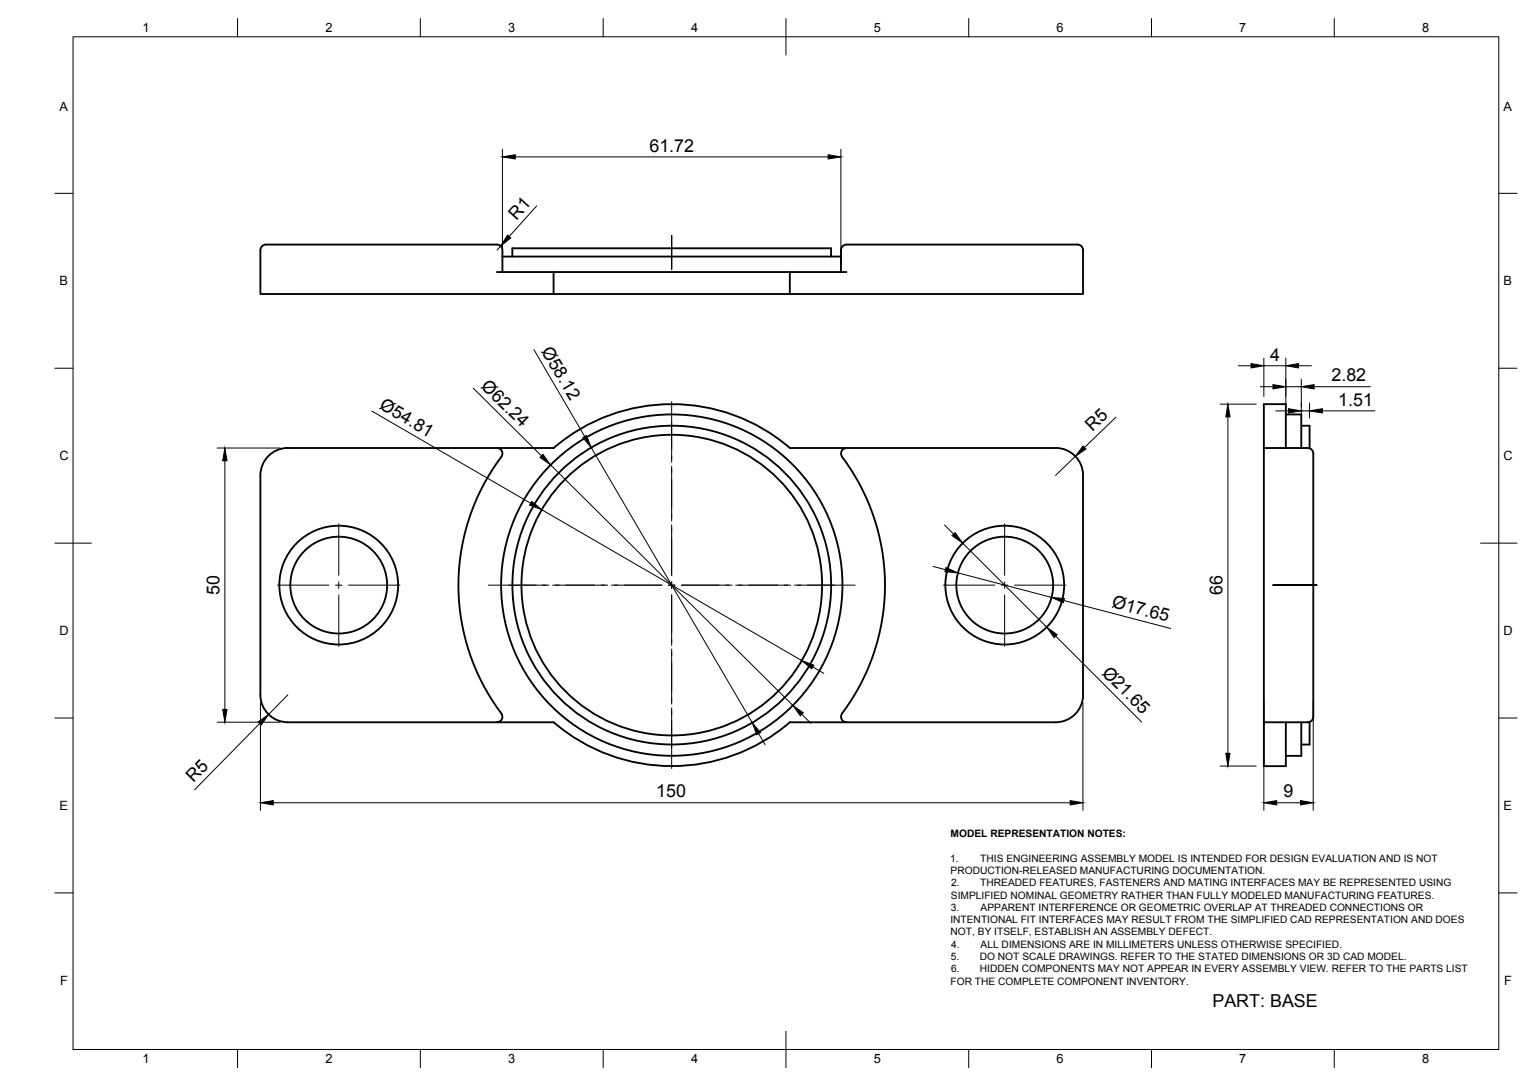
ISO-10303-21;
HEADER;
/* Generated by software containing ST-Developer
 * from STEP Tools, Inc. (www.steptools.com) 
 */

FILE_DESCRIPTION(
/* description */ (''),
/* implementation_level */ '2;1');

FILE_NAME(
/* name */ 'Base.step',
/* time_stamp */ '2026-10-04T22:47:03-07:00',
/* author */ (''),
/* organization */ (''),
/* preprocessor_version */ 'ST-DEVELOPER v20.2',
/* originating_system */ 'Autodesk Translation Framework v15.15.0.0',
/* authorisation */ '');

FILE_SCHEMA (('AUTOMOTIVE_DESIGN { 1 0 10303 214 3 1 1 }'));
ENDSEC;

DATA;
#10=MECHANICAL_DESIGN_GEOMETRIC_PRESENTATION_REPRESENTATION('',(#82),#19878);
#39=SPHERICAL_SURFACE('',#5318,1.);
#40=SPHERICAL_SURFACE('',#5323,1.);
#41=SPHERICAL_SURFACE('',#5367,1.);
#42=SPHERICAL_SURFACE('',#5372,1.);
#50=TOROIDAL_SURFACE('',#5313,39.889325151227,1.);
#51=TOROIDAL_SURFACE('',#5335,4.,1.);
#52=TOROIDAL_SURFACE('',#5340,4.,1.);
#53=TOROIDAL_SURFACE('',#5362,39.889325151227,1.);
#54=TOROIDAL_SURFACE('',#5384,4.,1.);
#55=TOROIDAL_SURFACE('',#5389,4.,1.);
#61=CONICAL_SURFACE('',#5342,9.8273485245745,0.785398163397449);
#62=CONICAL_SURFACE('',#5391,9.8273485245745,0.785398163397449);
#68=SHAPE_REPRESENTATION_RELATIONSHIP('SRR','None',#19912,#75);
#75=ADVANCED_BREP_SHAPE_REPRESENTATION('',(#89),#19876);
#82=STYLED_ITEM('',(#19951),#89);
#89=MANIFOLD_SOLID_BREP('Body1',#4830);
#104=FACE_BOUND('',#849,.T.);
#105=FACE_BOUND('',#871,.T.);
#106=FACE_BOUND('',#886,.T.);
#107=FACE_BOUND('',#887,.T.);
#108=FACE_BOUND('',#889,.T.);
#109=FACE_BOUND('',#892,.T.);
#110=FACE_BOUND('',#895,.T.);
#312=PLANE('',#5325);
#313=PLANE('',#5328);
#314=PLANE('',#5334);
#315=PLANE('',#5348);
#316=PLANE('',#5374);
#317=PLANE('',#5377);
#318=PLANE('',#5383);
#319=PLANE('',#5397);
#320=PLANE('',#5405);
#321=PLANE('',#5406);
#322=PLANE('',#5407);
#323=PLANE('',#5411);
#324=PLANE('',#5415);
#552=FACE_OUTER_BOUND('',#841,.T.);
#553=FACE_OUTER_BOUND('',#842,.T.);
#554=FACE_OUTER_BOUND('',#843,.T.);
#555=FACE_OUTER_BOUND('',#844,.T.);
#556=FACE_OUTER_BOUND('',#845,.T.);
#557=FACE_OUTER_BOUND('',#846,.T.);
#558=FACE_OUTER_BOUND('',#847,.T.);
#559=FACE_OUTER_BOUND('',#848,.T.);
#560=FACE_OUTER_BOUND('',#850,.T.);
#561=FACE_OUTER_BOUND('',#851,.T.);
#562=FACE_OUTER_BOUND('',#852,.T.);
#563=FACE_OUTER_BOUND('',#853,.T.);
#564=FACE_OUTER_BOUND('',#854,.T.);
#565=FACE_OUTER_BOUND('',#855,.T.);
#566=FACE_OUTER_BOUND('',#856,.T.);
#567=FACE_OUTER_BOUND('',#857,.T.);
#568=FACE_OUTER_BOUND('',#858,.T.);
#569=FACE_OUTER_BOUND('',#859,.T.);
#570=FACE_OUTER_BOUND('',#860,.T.);
#571=FACE_OUTER_BOUND('',#861,.T.);
#572=FACE_OUTER_BOUND('',#862,.T.);
#573=FACE_OUTER_BOUND('',#863,.T.);
#574=FACE_OUTER_BOUND('',#864,.T.);
#575=FACE_OUTER_BOUND('',#865,.T.);
#576=FACE_OUTER_BOUND('',#866,.T.);
#577=FACE_OUTER_BOUND('',#867,.T.);
#578=FACE_OUTER_BOUND('',#868,.T.);
#579=FACE_OUTER_BOUND('',#869,.T.);
#580=FACE_OUTER_BOUND('',#870,.T.);
#581=FACE_OUTER_BOUND('',#872,.T.);
#582=FACE_OUTER_BOUND('',#873,.T.);
#583=FACE_OUTER_BOUND('',#874,.T.);
#584=FACE_OUTER_BOUND('',#875,.T.);
#585=FACE_OUTER_BOUND('',#876,.T.);
#586=FACE_OUTER_BOUND('',#877,.T.);
#587=FACE_OUTER_BOUND('',#878,.T.);
#588=FACE_OUTER_BOUND('',#879,.T.);
#589=FACE_OUTER_BOUND('',#880,.T.);
#590=FACE_OUTER_BOUND('',#881,.T.);
#591=FACE_OUTER_BOUND('',#882,.T.);
#592=FACE_OUTER_BOUND('',#883,.T.);
#593=FACE_OUTER_BOUND('',#884,.T.);
#594=FACE_OUTER_BOUND('',#885,.T.);
#595=FACE_OUTER_BOUND('',#888,.T.);
#596=FACE_OUTER_BOUND('',#890,.T.);
#597=FACE_OUTER_BOUND('',#891,.T.);
#598=FACE_OUTER_BOUND('',#893,.T.);
#599=FACE_OUTER_BOUND('',#894,.T.);
#841=EDGE_LOOP('',(#4213,#4214,#4215,#4216));
#842=EDGE_LOOP('',(#4217,#4218,#4219,#4220));
#843=EDGE_LOOP('',(#4221,#4222,#4223));
#844=EDGE_LOOP('',(#4224,#4225,#4226,#4227));
#845=EDGE_LOOP('',(#4228,#4229,#4230));
#846=EDGE_LOOP('',(#4231,#4232,#4233,#4234,#4235,#4236));
#847=EDGE_LOOP('',(#4237,#4238,#4239,#4240));
#848=EDGE_LOOP('',(#4241,#4242,#4243,#4244,#4245,#4246));
#849=EDGE_LOOP('',(#4247));
#850=EDGE_LOOP('',(#4248,#4249,#4250,#4251));
#851=EDGE_LOOP('',(#4252,#4253,#4254,#4255,#4256,#4257));
#852=EDGE_LOOP('',(#4258,#4259,#4260,#4261));
#853=EDGE_LOOP('',(#4262,#4263,#4264,#4265));
#854=EDGE_LOOP('',(#4266,#4267,#4268,#4269));
#855=EDGE_LOOP('',(#4270,#4271,#4272,#4273));
#856=EDGE_LOOP('',(#4274,#4275,#4276,#4277));
#857=EDGE_LOOP('',(#4278,#4279,#4280,#4281));
#858=EDGE_LOOP('',(#4282,#4283,#4284,#4285));
#859=EDGE_LOOP('',(#4286,#4287,#4288,#4289));
#860=EDGE_LOOP('',(#4290,#4291,#4292,#4293));
#861=EDGE_LOOP('',(#4294,#4295,#4296,#4297));
#862=EDGE_LOOP('',(#4298,#4299,#4300,#4301));
#863=EDGE_LOOP('',(#4302,#4303,#4304,#4305));
#864=EDGE_LOOP('',(#4306,#4307,#4308,#4309));
#865=EDGE_LOOP('',(#4310,#4311,#4312));
#866=EDGE_LOOP('',(#4313,#4314,#4315,#4316));
#867=EDGE_LOOP('',(#4317,#4318,#4319));
#868=EDGE_LOOP('',(#4320,#4321,#4322,#4323,#4324,#4325));
#869=EDGE_LOOP('',(#4326,#4327,#4328,#4329));
#870=EDGE_LOOP('',(#4330,#4331,#4332,#4333,#4334,#4335));
#871=EDGE_LOOP('',(#4336));
#872=EDGE_LOOP('',(#4337,#4338,#4339,#4340));
#873=EDGE_LOOP('',(#4341,#4342,#4343,#4344,#4345,#4346));
#874=EDGE_LOOP('',(#4347,#4348,#4349,#4350));
#875=EDGE_LOOP('',(#4351,#4352,#4353,#4354));
#876=EDGE_LOOP('',(#4355,#4356,#4357,#4358));
#877=EDGE_LOOP('',(#4359,#4360,#4361,#4362));
#878=EDGE_LOOP('',(#4363,#4364,#4365,#4366));
#879=EDGE_LOOP('',(#4367,#4368,#4369,#4370));
#880=EDGE_LOOP('',(#4371,#4372,#4373,#4374));
#881=EDGE_LOOP('',(#4375,#4376,#4377,#4378));
#882=EDGE_LOOP('',(#4379,#4380,#4381,#4382));
#883=EDGE_LOOP('',(#4383,#4384,#4385,#4386));
#884=EDGE_LOOP('',(#4387));
#885=EDGE_LOOP('',(#4388,#4389,#4390,#4391,#4392,#4393,#4394,#4395,#4396,
#4397,#4398,#4399));
#886=EDGE_LOOP('',(#4400));
#887=EDGE_LOOP('',(#4401));
#888=EDGE_LOOP('',(#4402,#4403,#4404,#4405,#4406,#4407,#4408,#4409,#4410,
#4411,#4412,#4413));
#889=EDGE_LOOP('',(#4414));
#890=EDGE_LOOP('',(#4415,#4416,#4417,#4418));
#891=EDGE_LOOP('',(#4419));
#892=EDGE_LOOP('',(#4420));
#893=EDGE_LOOP('',(#4421,#4422,#4423,#4424));
#894=EDGE_LOOP('',(#4425));
#895=EDGE_LOOP('',(#4426));
#1204=LINE('',#19635,#1560);
#1205=LINE('',#19638,#1561);
#1206=LINE('',#19653,#1562);
#1207=LINE('',#19656,#1563);
#1208=LINE('',#19661,#1564);
#1209=LINE('',#19663,#1565);
#1210=LINE('',#19665,#1566);
#1211=LINE('',#19667,#1567);
#1212=LINE('',#19668,#1568);
#1213=LINE('',#19672,#1569);
#1214=LINE('',#19677,#1570);
#1215=LINE('',#19680,#1571);
#1216=LINE('',#19686,#1572);
#1217=LINE('',#19689,#1573);
#1218=LINE('',#19691,#1574);
#1219=LINE('',#19693,#1575);
#1220=LINE('',#19694,#1576);
#1221=LINE('',#19702,#1577);
#1222=LINE('',#19708,#1578);
#1223=LINE('',#19712,#1579);
#1224=LINE('',#19716,#1580);
#1225=LINE('',#19719,#1581);
#1226=LINE('',#19720,#1582);
#1227=LINE('',#19729,#1583);
#1228=LINE('',#19735,#1584);
#1229=LINE('',#19742,#1585);
#1230=LINE('',#19745,#1586);
#1231=LINE('',#19760,#1587);
#1232=LINE('',#19763,#1588);
#1233=LINE('',#19767,#1589);
#1234=LINE('',#19769,#1590);
#1235=LINE('',#19771,#1591);
#1236=LINE('',#19772,#1592);
#1237=LINE('',#19775,#1593);
#1238=LINE('',#19779,#1594);
#1239=LINE('',#19783,#1595);
#1240=LINE('',#19789,#1596);
#1241=LINE('',#19792,#1597);
#1242=LINE('',#19794,#1598);
#1243=LINE('',#19795,#1599);
#1244=LINE('',#19803,#1600);
#1245=LINE('',#19809,#1601);
#1246=LINE('',#19812,#1602);
#1247=LINE('',#19816,#1603);
#1248=LINE('',#19820,#1604);
#1249=LINE('',#19821,#1605);
#1250=LINE('',#19830,#1606);
#1251=LINE('',#19840,#1607);
#1252=LINE('',#19847,#1608);
#1560=VECTOR('',#6538,10.);
#1561=VECTOR('',#6541,10.);
#1562=VECTOR('',#6560,10.);
#1563=VECTOR('',#6563,10.);
#1564=VECTOR('',#6570,10.);
#1565=VECTOR('',#6571,10.);
#1566=VECTOR('',#6572,10.);
#1567=VECTOR('',#6573,10.);
#1568=VECTOR('',#6574,10.);
#1569=VECTOR('',#6579,10.);
#1570=VECTOR('',#6584,10.);
#1571=VECTOR('',#6587,10.);
#1572=VECTOR('',#6594,10.);
#1573=VECTOR('',#6597,10.);
#1574=VECTOR('',#6598,10.);
#1575=VECTOR('',#6599,10.);
#1576=VECTOR('',#6600,10.);
#1577=VECTOR('',#6611,10.);
#1578=VECTOR('',#6620,9.8273485245745);
#1579=VECTOR('',#6625,8.8273485245745);
#1580=VECTOR('',#6630,10.);
#1581=VECTOR('',#6633,10.);
#1582=VECTOR('',#6634,10.);
#1583=VECTOR('',#6647,10.);
#1584=VECTOR('',#6654,10.);
#1585=VECTOR('',#6661,10.);
#1586=VECTOR('',#6664,10.);
#1587=VECTOR('',#6683,10.);
#1588=VECTOR('',#6686,10.);
#1589=VECTOR('',#6693,10.);
#1590=VECTOR('',#6694,10.);
#1591=VECTOR('',#6695,10.);
#1592=VECTOR('',#6696,10.);
#1593=VECTOR('',#6699,10.);
#1594=VECTOR('',#6704,10.);
#1595=VECTOR('',#6707,10.);
#1596=VECTOR('',#6714,10.);
#1597=VECTOR('',#6719,10.);
#1598=VECTOR('',#6720,10.);
#1599=VECTOR('',#6721,10.);
#1600=VECTOR('',#6732,10.);
#1601=VECTOR('',#6741,9.8273485245745);
#1602=VECTOR('',#6744,8.8273485245745);
#1603=VECTOR('',#6749,10.);
#1604=VECTOR('',#6754,10.);
#1605=VECTOR('',#6755,10.);
#1606=VECTOR('',#6768,27.4027293621977);
#1607=VECTOR('',#6783,31.1192710879259);
#1608=VECTOR('',#6792,29.0578798664922);
#1815=CIRCLE('',#5311,0.999999999999996);
#1816=CIRCLE('',#5312,1.);
#1817=CIRCLE('',#5314,0.999999999999999);
#1818=CIRCLE('',#5315,38.889325151227);
#1819=CIRCLE('',#5316,1.);
#1820=CIRCLE('',#5317,39.889325151227);
#1821=CIRCLE('',#5319,1.);
#1822=CIRCLE('',#5321,1.);
#1823=CIRCLE('',#5322,1.);
#1824=CIRCLE('',#5324,1.);
#1825=CIRCLE('',#5327,1.);
#1826=CIRCLE('',#5329,4.);
#1827=CIRCLE('',#5330,4.);
#1828=CIRCLE('',#5331,10.8273485245745);
#1829=CIRCLE('',#5333,1.);
#1830=CIRCLE('',#5336,1.);
#1831=CIRCLE('',#5337,5.);
#1832=CIRCLE('',#5339,1.);
#1833=CIRCLE('',#5341,5.);
#1834=CIRCLE('',#5343,8.8273485245745);
#1835=CIRCLE('',#5345,8.8273485245745);
#1836=CIRCLE('',#5347,5.);
#1837=CIRCLE('',#5350,5.);
#1838=CIRCLE('',#5352,38.889325151227);
#1839=CIRCLE('',#5354,33.);
#1840=CIRCLE('',#5355,33.);
#1841=CIRCLE('',#5357,33.);
#1842=CIRCLE('',#5358,33.);
#1843=CIRCLE('',#5360,0.999999999999996);
#1844=CIRCLE('',#5361,1.);
#1845=CIRCLE('',#5363,0.999999999999999);
#1846=CIRCLE('',#5364,39.889325151227);
#1847=CIRCLE('',#5365,1.);
#1848=CIRCLE('',#5366,38.889325151227);
#1849=CIRCLE('',#5368,1.);
#1850=CIRCLE('',#5370,1.);
#1851=CIRCLE('',#5371,1.);
#1852=CIRCLE('',#5373,1.);
#1853=CIRCLE('',#5376,1.);
#1854=CIRCLE('',#5378,4.);
#1855=CIRCLE('',#5379,4.);
#1856=CIRCLE('',#5380,10.8273485245745);
#1857=CIRCLE('',#5382,1.);
#1858=CIRCLE('',#5385,1.);
#1859=CIRCLE('',#5386,5.);
#1860=CIRCLE('',#5388,1.);
#1861=CIRCLE('',#5390,5.);
#1862=CIRCLE('',#5392,8.8273485245745);
#1863=CIRCLE('',#5394,8.8273485245745);
#1864=CIRCLE('',#5396,5.);
#1865=CIRCLE('',#5399,5.);
#1866=CIRCLE('',#5401,38.889325151227);
#1867=CIRCLE('',#5403,27.4027293621977);
#1868=CIRCLE('',#5404,27.4027293621977);
#1869=CIRCLE('',#5408,31.1192710879259);
#1870=CIRCLE('',#5410,31.1192710879259);
#1871=CIRCLE('',#5412,29.0578798664922);
#1872=CIRCLE('',#5414,29.0578798664922);
#2260=VERTEX_POINT('',#19631);
#2261=VERTEX_POINT('',#19632);
#2262=VERTEX_POINT('',#19634);
#2263=VERTEX_POINT('',#19636);
#2264=VERTEX_POINT('',#19640);
#2265=VERTEX_POINT('',#19641);
#2266=VERTEX_POINT('',#19644);
#2267=VERTEX_POINT('',#19650);
#2268=VERTEX_POINT('',#19652);
#2269=VERTEX_POINT('',#19654);
#2270=VERTEX_POINT('',#19660);
#2271=VERTEX_POINT('',#19662);
#2272=VERTEX_POINT('',#19664);
#2273=VERTEX_POINT('',#19666);
#2274=VERTEX_POINT('',#19670);
#2275=VERTEX_POINT('',#19674);
#2276=VERTEX_POINT('',#19676);
#2277=VERTEX_POINT('',#19678);
#2278=VERTEX_POINT('',#19681);
#2279=VERTEX_POINT('',#19684);
#2280=VERTEX_POINT('',#19688);
#2281=VERTEX_POINT('',#19690);
#2282=VERTEX_POINT('',#19692);
#2283=VERTEX_POINT('',#19696);
#2284=VERTEX_POINT('',#19700);
#2285=VERTEX_POINT('',#19706);
#2286=VERTEX_POINT('',#19710);
#2287=VERTEX_POINT('',#19714);
#2288=VERTEX_POINT('',#19718);
#2289=VERTEX_POINT('',#19726);
#2290=VERTEX_POINT('',#19728);
#2291=VERTEX_POINT('',#19732);
#2292=VERTEX_POINT('',#19734);
#2293=VERTEX_POINT('',#19738);
#2294=VERTEX_POINT('',#19739);
#2295=VERTEX_POINT('',#19741);
#2296=VERTEX_POINT('',#19743);
#2297=VERTEX_POINT('',#19747);
#2298=VERTEX_POINT('',#19748);
#2299=VERTEX_POINT('',#19750);
#2300=VERTEX_POINT('',#19757);
#2301=VERTEX_POINT('',#19759);
#2302=VERTEX_POINT('',#19761);
#2303=VERTEX_POINT('',#19768);
#2304=VERTEX_POINT('',#19770);
#2305=VERTEX_POINT('',#19774);
#2306=VERTEX_POINT('',#19778);
#2307=VERTEX_POINT('',#19780);
#2308=VERTEX_POINT('',#19782);
#2309=VERTEX_POINT('',#19785);
#2310=VERTEX_POINT('',#19788);
#2311=VERTEX_POINT('',#19793);
#2312=VERTEX_POINT('',#19797);
#2313=VERTEX_POINT('',#19801);
#2314=VERTEX_POINT('',#19807);
#2315=VERTEX_POINT('',#19811);
#2316=VERTEX_POINT('',#19815);
#2317=VERTEX_POINT('',#19819);
#2318=VERTEX_POINT('',#19827);
#2319=VERTEX_POINT('',#19829);
#2320=VERTEX_POINT('',#19835);
#2321=VERTEX_POINT('',#19838);
#2322=VERTEX_POINT('',#19842);
#2323=VERTEX_POINT('',#19845);
#2918=EDGE_CURVE('',#2260,#2261,#1815,.T.);
#2919=EDGE_CURVE('',#2262,#2260,#1204,.T.);
#2920=EDGE_CURVE('',#2263,#2262,#1816,.F.);
#2921=EDGE_CURVE('',#2261,#2263,#1205,.T.);
#2922=EDGE_CURVE('',#2264,#2265,#1817,.T.);
#2923=EDGE_CURVE('',#2260,#2264,#1818,.T.);
#2924=EDGE_CURVE('',#2266,#2260,#1819,.T.);
#2925=EDGE_CURVE('',#2265,#2266,#1820,.T.);
#2926=EDGE_CURVE('',#2266,#2261,#1821,.T.);
#2927=EDGE_CURVE('',#2267,#2264,#1822,.T.);
#2928=EDGE_CURVE('',#2268,#2267,#1206,.T.);
#2929=EDGE_CURVE('',#2269,#2268,#1823,.F.);
#2930=EDGE_CURVE('',#2264,#2269,#1207,.T.);
#2931=EDGE_CURVE('',#2267,#2265,#1824,.T.);
#2932=EDGE_CURVE('',#2270,#2263,#1208,.T.);
#2933=EDGE_CURVE('',#2271,#2270,#1209,.T.);
#2934=EDGE_CURVE('',#2271,#2272,#1210,.T.);
#2935=EDGE_CURVE('',#2272,#2273,#1211,.T.);
#2936=EDGE_CURVE('',#2273,#2261,#1212,.T.);
#2937=EDGE_CURVE('',#2274,#2273,#1825,.T.);
#2938=EDGE_CURVE('',#2266,#2274,#1213,.T.);
#2939=EDGE_CURVE('',#2274,#2275,#1826,.T.);
#2940=EDGE_CURVE('',#2275,#2276,#1214,.T.);
#2941=EDGE_CURVE('',#2276,#2277,#1827,.T.);
#2942=EDGE_CURVE('',#2277,#2265,#1215,.T.);
#2943=EDGE_CURVE('',#2278,#2278,#1828,.T.);
#2944=EDGE_CURVE('',#2277,#2279,#1829,.T.);
#2945=EDGE_CURVE('',#2267,#2279,#1216,.T.);
#2946=EDGE_CURVE('',#2279,#2280,#1217,.T.);
#2947=EDGE_CURVE('',#2280,#2281,#1218,.T.);
#2948=EDGE_CURVE('',#2282,#2281,#1219,.T.);
#2949=EDGE_CURVE('',#2268,#2282,#1220,.T.);
#2950=EDGE_CURVE('',#2275,#2283,#1830,.T.);
#2951=EDGE_CURVE('',#2283,#2273,#1831,.T.);
#2952=EDGE_CURVE('',#2276,#2284,#1832,.T.);
#2953=EDGE_CURVE('',#2284,#2283,#1221,.T.);
#2954=EDGE_CURVE('',#2279,#2284,#1833,.T.);
#2955=EDGE_CURVE('',#2285,#2285,#1834,.T.);
#2956=EDGE_CURVE('',#2285,#2278,#1222,.T.);
#2957=EDGE_CURVE('',#2286,#2286,#1835,.T.);
#2958=EDGE_CURVE('',#2286,#2285,#1223,.T.);
#2959=EDGE_CURVE('',#2287,#2272,#1836,.T.);
#2960=EDGE_CURVE('',#2283,#2287,#1224,.T.);
#2961=EDGE_CURVE('',#2287,#2288,#1225,.T.);
#2962=EDGE_CURVE('',#2288,#2284,#1226,.T.);
#2963=EDGE_CURVE('',#2280,#2288,#1837,.T.);
#2964=EDGE_CURVE('',#2262,#2269,#1838,.T.);
#2965=EDGE_CURVE('',#2281,#2289,#1839,.F.);
#2966=EDGE_CURVE('',#2289,#2290,#1227,.T.);
#2967=EDGE_CURVE('',#2282,#2290,#1840,.T.);
#2968=EDGE_CURVE('',#2291,#2270,#1841,.T.);
#2969=EDGE_CURVE('',#2291,#2292,#1228,.T.);
#2970=EDGE_CURVE('',#2292,#2271,#1842,.F.);
#2971=EDGE_CURVE('',#2293,#2294,#1843,.T.);
#2972=EDGE_CURVE('',#2294,#2295,#1229,.T.);
#2973=EDGE_CURVE('',#2295,#2296,#1844,.F.);
#2974=EDGE_CURVE('',#2296,#2293,#1230,.T.);
#2975=EDGE_CURVE('',#2297,#2298,#1845,.T.);
#2976=EDGE_CURVE('',#2298,#2299,#1846,.T.);
#2977=EDGE_CURVE('',#2299,#2293,#1847,.T.);
#2978=EDGE_CURVE('',#2293,#2297,#1848,.T.);
#2979=EDGE_CURVE('',#2299,#2294,#1849,.T.);
#2980=EDGE_CURVE('',#2300,#2297,#1850,.T.);
#2981=EDGE_CURVE('',#2297,#2301,#1231,.T.);
#2982=EDGE_CURVE('',#2301,#2302,#1851,.F.);
#2983=EDGE_CURVE('',#2302,#2300,#1232,.T.);
#2984=EDGE_CURVE('',#2300,#2298,#1852,.T.);
#2985=EDGE_CURVE('',#2291,#2295,#1233,.T.);
#2986=EDGE_CURVE('',#2303,#2294,#1234,.T.);
#2987=EDGE_CURVE('',#2304,#2303,#1235,.T.);
#2988=EDGE_CURVE('',#2292,#2304,#1236,.T.);
#2989=EDGE_CURVE('',#2299,#2305,#1237,.T.);
#2990=EDGE_CURVE('',#2305,#2303,#1853,.T.);
#2991=EDGE_CURVE('',#2306,#2298,#1238,.T.);
#2992=EDGE_CURVE('',#2307,#2306,#1854,.T.);
#2993=EDGE_CURVE('',#2308,#2307,#1239,.T.);
#2994=EDGE_CURVE('',#2305,#2308,#1855,.T.);
#2995=EDGE_CURVE('',#2309,#2309,#1856,.T.);
#2996=EDGE_CURVE('',#2300,#2310,#1240,.T.);
#2997=EDGE_CURVE('',#2306,#2310,#1857,.T.);
#2998=EDGE_CURVE('',#2302,#2290,#1241,.T.);
#2999=EDGE_CURVE('',#2311,#2289,#1242,.T.);
#3000=EDGE_CURVE('',#2310,#2311,#1243,.T.);
#3001=EDGE_CURVE('',#2308,#2312,#1858,.T.);
#3002=EDGE_CURVE('',#2312,#2303,#1859,.T.);
#3003=EDGE_CURVE('',#2307,#2313,#1860,.T.);
#3004=EDGE_CURVE('',#2313,#2312,#1244,.T.);
#3005=EDGE_CURVE('',#2310,#2313,#1861,.T.);
#3006=EDGE_CURVE('',#2314,#2314,#1862,.T.);
#3007=EDGE_CURVE('',#2314,#2309,#1245,.T.);
#3008=EDGE_CURVE('',#2314,#2315,#1246,.T.);
#3009=EDGE_CURVE('',#2315,#2315,#1863,.T.);
#3010=EDGE_CURVE('',#2312,#2316,#1247,.T.);
#3011=EDGE_CURVE('',#2316,#2304,#1864,.T.);
#3012=EDGE_CURVE('',#2317,#2313,#1248,.T.);
#3013=EDGE_CURVE('',#2316,#2317,#1249,.T.);
#3014=EDGE_CURVE('',#2311,#2317,#1865,.T.);
#3015=EDGE_CURVE('',#2296,#2301,#1866,.T.);
#3016=EDGE_CURVE('',#2318,#2318,#1867,.T.);
#3017=EDGE_CURVE('',#2318,#2319,#1250,.T.);
#3018=EDGE_CURVE('',#2319,#2319,#1868,.T.);
#3019=EDGE_CURVE('',#2320,#2320,#1869,.T.);
#3020=EDGE_CURVE('',#2321,#2321,#1870,.T.);
#3021=EDGE_CURVE('',#2321,#2320,#1251,.T.);
#3022=EDGE_CURVE('',#2322,#2322,#1871,.T.);
#3023=EDGE_CURVE('',#2323,#2323,#1872,.T.);
#3024=EDGE_CURVE('',#2323,#2322,#1252,.T.);
#4213=ORIENTED_EDGE('',*,*,#2918,.F.);
#4214=ORIENTED_EDGE('',*,*,#2919,.F.);
#4215=ORIENTED_EDGE('',*,*,#2920,.F.);
#4216=ORIENTED_EDGE('',*,*,#2921,.F.);
#4217=ORIENTED_EDGE('',*,*,#2922,.F.);
#4218=ORIENTED_EDGE('',*,*,#2923,.F.);
#4219=ORIENTED_EDGE('',*,*,#2924,.F.);
#4220=ORIENTED_EDGE('',*,*,#2925,.F.);
#4221=ORIENTED_EDGE('',*,*,#2924,.T.);
#4222=ORIENTED_EDGE('',*,*,#2918,.T.);
#4223=ORIENTED_EDGE('',*,*,#2926,.F.);
#4224=ORIENTED_EDGE('',*,*,#2927,.F.);
#4225=ORIENTED_EDGE('',*,*,#2928,.F.);
#4226=ORIENTED_EDGE('',*,*,#2929,.F.);
#4227=ORIENTED_EDGE('',*,*,#2930,.F.);
#4228=ORIENTED_EDGE('',*,*,#2927,.T.);
#4229=ORIENTED_EDGE('',*,*,#2922,.T.);
#4230=ORIENTED_EDGE('',*,*,#2931,.F.);
#4231=ORIENTED_EDGE('',*,*,#2932,.F.);
#4232=ORIENTED_EDGE('',*,*,#2933,.F.);
#4233=ORIENTED_EDGE('',*,*,#2934,.T.);
#4234=ORIENTED_EDGE('',*,*,#2935,.T.);
#4235=ORIENTED_EDGE('',*,*,#2936,.T.);
#4236=ORIENTED_EDGE('',*,*,#2921,.T.);
#4237=ORIENTED_EDGE('',*,*,#2926,.T.);
#4238=ORIENTED_EDGE('',*,*,#2936,.F.);
#4239=ORIENTED_EDGE('',*,*,#2937,.F.);
#4240=ORIENTED_EDGE('',*,*,#2938,.F.);
#4241=ORIENTED_EDGE('',*,*,#2925,.T.);
#4242=ORIENTED_EDGE('',*,*,#2938,.T.);
#4243=ORIENTED_EDGE('',*,*,#2939,.T.);
#4244=ORIENTED_EDGE('',*,*,#2940,.T.);
#4245=ORIENTED_EDGE('',*,*,#2941,.T.);
#4246=ORIENTED_EDGE('',*,*,#2942,.T.);
#4247=ORIENTED_EDGE('',*,*,#2943,.T.);
#4248=ORIENTED_EDGE('',*,*,#2931,.T.);
#4249=ORIENTED_EDGE('',*,*,#2942,.F.);
#4250=ORIENTED_EDGE('',*,*,#2944,.T.);
#4251=ORIENTED_EDGE('',*,*,#2945,.F.);
#4252=ORIENTED_EDGE('',*,*,#2928,.T.);
#4253=ORIENTED_EDGE('',*,*,#2945,.T.);
#4254=ORIENTED_EDGE('',*,*,#2946,.T.);
#4255=ORIENTED_EDGE('',*,*,#2947,.T.);
#4256=ORIENTED_EDGE('',*,*,#2948,.F.);
#4257=ORIENTED_EDGE('',*,*,#2949,.F.);
#4258=ORIENTED_EDGE('',*,*,#2950,.F.);
#4259=ORIENTED_EDGE('',*,*,#2939,.F.);
#4260=ORIENTED_EDGE('',*,*,#2937,.T.);
#4261=ORIENTED_EDGE('',*,*,#2951,.F.);
#4262=ORIENTED_EDGE('',*,*,#2952,.F.);
#4263=ORIENTED_EDGE('',*,*,#2940,.F.);
#4264=ORIENTED_EDGE('',*,*,#2950,.T.);
#4265=ORIENTED_EDGE('',*,*,#2953,.F.);
#4266=ORIENTED_EDGE('',*,*,#2944,.F.);
#4267=ORIENTED_EDGE('',*,*,#2941,.F.);
#4268=ORIENTED_EDGE('',*,*,#2952,.T.);
#4269=ORIENTED_EDGE('',*,*,#2954,.F.);
#4270=ORIENTED_EDGE('',*,*,#2955,.F.);
#4271=ORIENTED_EDGE('',*,*,#2956,.T.);
#4272=ORIENTED_EDGE('',*,*,#2943,.F.);
#4273=ORIENTED_EDGE('',*,*,#2956,.F.);
#4274=ORIENTED_EDGE('',*,*,#2957,.T.);
#4275=ORIENTED_EDGE('',*,*,#2958,.T.);
#4276=ORIENTED_EDGE('',*,*,#2955,.T.);
#4277=ORIENTED_EDGE('',*,*,#2958,.F.);
#4278=ORIENTED_EDGE('',*,*,#2951,.T.);
#4279=ORIENTED_EDGE('',*,*,#2935,.F.);
#4280=ORIENTED_EDGE('',*,*,#2959,.F.);
#4281=ORIENTED_EDGE('',*,*,#2960,.F.);
#4282=ORIENTED_EDGE('',*,*,#2953,.T.);
#4283=ORIENTED_EDGE('',*,*,#2960,.T.);
#4284=ORIENTED_EDGE('',*,*,#2961,.T.);
#4285=ORIENTED_EDGE('',*,*,#2962,.T.);
#4286=ORIENTED_EDGE('',*,*,#2954,.T.);
#4287=ORIENTED_EDGE('',*,*,#2962,.F.);
#4288=ORIENTED_EDGE('',*,*,#2963,.F.);
#4289=ORIENTED_EDGE('',*,*,#2946,.F.);
#4290=ORIENTED_EDGE('',*,*,#2919,.T.);
#4291=ORIENTED_EDGE('',*,*,#2923,.T.);
#4292=ORIENTED_EDGE('',*,*,#2930,.T.);
#4293=ORIENTED_EDGE('',*,*,#2964,.F.);
#4294=ORIENTED_EDGE('',*,*,#2948,.T.);
#4295=ORIENTED_EDGE('',*,*,#2965,.T.);
#4296=ORIENTED_EDGE('',*,*,#2966,.T.);
#4297=ORIENTED_EDGE('',*,*,#2967,.F.);
#4298=ORIENTED_EDGE('',*,*,#2933,.T.);
#4299=ORIENTED_EDGE('',*,*,#2968,.F.);
#4300=ORIENTED_EDGE('',*,*,#2969,.T.);
#4301=ORIENTED_EDGE('',*,*,#2970,.T.);
#4302=ORIENTED_EDGE('',*,*,#2971,.T.);
#4303=ORIENTED_EDGE('',*,*,#2972,.T.);
#4304=ORIENTED_EDGE('',*,*,#2973,.T.);
#4305=ORIENTED_EDGE('',*,*,#2974,.T.);
#4306=ORIENTED_EDGE('',*,*,#2975,.T.);
#4307=ORIENTED_EDGE('',*,*,#2976,.T.);
#4308=ORIENTED_EDGE('',*,*,#2977,.T.);
#4309=ORIENTED_EDGE('',*,*,#2978,.T.);
#4310=ORIENTED_EDGE('',*,*,#2977,.F.);
#4311=ORIENTED_EDGE('',*,*,#2979,.T.);
#4312=ORIENTED_EDGE('',*,*,#2971,.F.);
#4313=ORIENTED_EDGE('',*,*,#2980,.T.);
#4314=ORIENTED_EDGE('',*,*,#2981,.T.);
#4315=ORIENTED_EDGE('',*,*,#2982,.T.);
#4316=ORIENTED_EDGE('',*,*,#2983,.T.);
#4317=ORIENTED_EDGE('',*,*,#2980,.F.);
#4318=ORIENTED_EDGE('',*,*,#2984,.T.);
#4319=ORIENTED_EDGE('',*,*,#2975,.F.);
#4320=ORIENTED_EDGE('',*,*,#2985,.T.);
#4321=ORIENTED_EDGE('',*,*,#2972,.F.);
#4322=ORIENTED_EDGE('',*,*,#2986,.F.);
#4323=ORIENTED_EDGE('',*,*,#2987,.F.);
#4324=ORIENTED_EDGE('',*,*,#2988,.F.);
#4325=ORIENTED_EDGE('',*,*,#2969,.F.);
#4326=ORIENTED_EDGE('',*,*,#2979,.F.);
#4327=ORIENTED_EDGE('',*,*,#2989,.T.);
#4328=ORIENTED_EDGE('',*,*,#2990,.T.);
#4329=ORIENTED_EDGE('',*,*,#2986,.T.);
#4330=ORIENTED_EDGE('',*,*,#2976,.F.);
#4331=ORIENTED_EDGE('',*,*,#2991,.F.);
#4332=ORIENTED_EDGE('',*,*,#2992,.F.);
#4333=ORIENTED_EDGE('',*,*,#2993,.F.);
#4334=ORIENTED_EDGE('',*,*,#2994,.F.);
#4335=ORIENTED_EDGE('',*,*,#2989,.F.);
#4336=ORIENTED_EDGE('',*,*,#2995,.F.);
#4337=ORIENTED_EDGE('',*,*,#2984,.F.);
#4338=ORIENTED_EDGE('',*,*,#2996,.T.);
#4339=ORIENTED_EDGE('',*,*,#2997,.F.);
#4340=ORIENTED_EDGE('',*,*,#2991,.T.);
#4341=ORIENTED_EDGE('',*,*,#2983,.F.);
#4342=ORIENTED_EDGE('',*,*,#2998,.T.);
#4343=ORIENTED_EDGE('',*,*,#2966,.F.);
#4344=ORIENTED_EDGE('',*,*,#2999,.F.);
#4345=ORIENTED_EDGE('',*,*,#3000,.F.);
#4346=ORIENTED_EDGE('',*,*,#2996,.F.);
#4347=ORIENTED_EDGE('',*,*,#3001,.T.);
#4348=ORIENTED_EDGE('',*,*,#3002,.T.);
#4349=ORIENTED_EDGE('',*,*,#2990,.F.);
#4350=ORIENTED_EDGE('',*,*,#2994,.T.);
#4351=ORIENTED_EDGE('',*,*,#3003,.T.);
#4352=ORIENTED_EDGE('',*,*,#3004,.T.);
#4353=ORIENTED_EDGE('',*,*,#3001,.F.);
#4354=ORIENTED_EDGE('',*,*,#2993,.T.);
#4355=ORIENTED_EDGE('',*,*,#2997,.T.);
#4356=ORIENTED_EDGE('',*,*,#3005,.T.);
#4357=ORIENTED_EDGE('',*,*,#3003,.F.);
#4358=ORIENTED_EDGE('',*,*,#2992,.T.);
#4359=ORIENTED_EDGE('',*,*,#3006,.T.);
#4360=ORIENTED_EDGE('',*,*,#3007,.T.);
#4361=ORIENTED_EDGE('',*,*,#2995,.T.);
#4362=ORIENTED_EDGE('',*,*,#3007,.F.);
#4363=ORIENTED_EDGE('',*,*,#3006,.F.);
#4364=ORIENTED_EDGE('',*,*,#3008,.T.);
#4365=ORIENTED_EDGE('',*,*,#3009,.F.);
#4366=ORIENTED_EDGE('',*,*,#3008,.F.);
#4367=ORIENTED_EDGE('',*,*,#3002,.F.);
#4368=ORIENTED_EDGE('',*,*,#3010,.T.);
#4369=ORIENTED_EDGE('',*,*,#3011,.T.);
#4370=ORIENTED_EDGE('',*,*,#2987,.T.);
#4371=ORIENTED_EDGE('',*,*,#3004,.F.);
#4372=ORIENTED_EDGE('',*,*,#3012,.F.);
#4373=ORIENTED_EDGE('',*,*,#3013,.F.);
#4374=ORIENTED_EDGE('',*,*,#3010,.F.);
#4375=ORIENTED_EDGE('',*,*,#3005,.F.);
#4376=ORIENTED_EDGE('',*,*,#3000,.T.);
#4377=ORIENTED_EDGE('',*,*,#3014,.T.);
#4378=ORIENTED_EDGE('',*,*,#3012,.T.);
#4379=ORIENTED_EDGE('',*,*,#2974,.F.);
#4380=ORIENTED_EDGE('',*,*,#3015,.T.);
#4381=ORIENTED_EDGE('',*,*,#2981,.F.);
#4382=ORIENTED_EDGE('',*,*,#2978,.F.);
#4383=ORIENTED_EDGE('',*,*,#3016,.F.);
#4384=ORIENTED_EDGE('',*,*,#3017,.T.);
#4385=ORIENTED_EDGE('',*,*,#3018,.T.);
#4386=ORIENTED_EDGE('',*,*,#3017,.F.);
#4387=ORIENTED_EDGE('',*,*,#3016,.T.);
#4388=ORIENTED_EDGE('',*,*,#2988,.T.);
#4389=ORIENTED_EDGE('',*,*,#3011,.F.);
#4390=ORIENTED_EDGE('',*,*,#3013,.T.);
#4391=ORIENTED_EDGE('',*,*,#3014,.F.);
#4392=ORIENTED_EDGE('',*,*,#2999,.T.);
#4393=ORIENTED_EDGE('',*,*,#2965,.F.);
#4394=ORIENTED_EDGE('',*,*,#2947,.F.);
#4395=ORIENTED_EDGE('',*,*,#2963,.T.);
#4396=ORIENTED_EDGE('',*,*,#2961,.F.);
#4397=ORIENTED_EDGE('',*,*,#2959,.T.);
#4398=ORIENTED_EDGE('',*,*,#2934,.F.);
#4399=ORIENTED_EDGE('',*,*,#2970,.F.);
#4400=ORIENTED_EDGE('',*,*,#2957,.F.);
#4401=ORIENTED_EDGE('',*,*,#3009,.T.);
#4402=ORIENTED_EDGE('',*,*,#2968,.T.);
#4403=ORIENTED_EDGE('',*,*,#2932,.T.);
#4404=ORIENTED_EDGE('',*,*,#2920,.T.);
#4405=ORIENTED_EDGE('',*,*,#2964,.T.);
#4406=ORIENTED_EDGE('',*,*,#2929,.T.);
#4407=ORIENTED_EDGE('',*,*,#2949,.T.);
#4408=ORIENTED_EDGE('',*,*,#2967,.T.);
#4409=ORIENTED_EDGE('',*,*,#2998,.F.);
#4410=ORIENTED_EDGE('',*,*,#2982,.F.);
#4411=ORIENTED_EDGE('',*,*,#3015,.F.);
#4412=ORIENTED_EDGE('',*,*,#2973,.F.);
#4413=ORIENTED_EDGE('',*,*,#2985,.F.);
#4414=ORIENTED_EDGE('',*,*,#3019,.F.);
#4415=ORIENTED_EDGE('',*,*,#3020,.F.);
#4416=ORIENTED_EDGE('',*,*,#3021,.T.);
#4417=ORIENTED_EDGE('',*,*,#3019,.T.);
#4418=ORIENTED_EDGE('',*,*,#3021,.F.);
#4419=ORIENTED_EDGE('',*,*,#3020,.T.);
#4420=ORIENTED_EDGE('',*,*,#3022,.F.);
#4421=ORIENTED_EDGE('',*,*,#3023,.F.);
#4422=ORIENTED_EDGE('',*,*,#3024,.T.);
#4423=ORIENTED_EDGE('',*,*,#3022,.T.);
#4424=ORIENTED_EDGE('',*,*,#3024,.F.);
#4425=ORIENTED_EDGE('',*,*,#3023,.T.);
#4426=ORIENTED_EDGE('',*,*,#3018,.F.);
#4526=CYLINDRICAL_SURFACE('',#5310,1.);
#4527=CYLINDRICAL_SURFACE('',#5320,1.);
#4528=CYLINDRICAL_SURFACE('',#5326,1.);
#4529=CYLINDRICAL_SURFACE('',#5332,1.);
#4530=CYLINDRICAL_SURFACE('',#5338,1.);
#4531=CYLINDRICAL_SURFACE('',#5344,8.8273485245745);
#4532=CYLINDRICAL_SURFACE('',#5346,5.);
#4533=CYLINDRICAL_SURFACE('',#5349,5.);
#4534=CYLINDRICAL_SURFACE('',#5351,38.889325151227);
#4535=CYLINDRICAL_SURFACE('',#5353,33.);
#4536=CYLINDRICAL_SURFACE('',#5356,33.);
#4537=CYLINDRICAL_SURFACE('',#5359,1.);
#4538=CYLINDRICAL_SURFACE('',#5369,1.);
#4539=CYLINDRICAL_SURFACE('',#5375,1.);
#4540=CYLINDRICAL_SURFACE('',#5381,1.);
#4541=CYLINDRICAL_SURFACE('',#5387,1.);
#4542=CYLINDRICAL_SURFACE('',#5393,8.8273485245745);
#4543=CYLINDRICAL_SURFACE('',#5395,5.);
#4544=CYLINDRICAL_SURFACE('',#5398,5.);
#4545=CYLINDRICAL_SURFACE('',#5400,38.889325151227);
#4546=CYLINDRICAL_SURFACE('',#5402,27.4027293621977);
#4547=CYLINDRICAL_SURFACE('',#5409,31.1192710879259);
#4548=CYLINDRICAL_SURFACE('',#5413,29.0578798664922);
#4776=ADVANCED_FACE('',(#552),#4526,.T.);
#4777=ADVANCED_FACE('',(#553),#50,.T.);
#4778=ADVANCED_FACE('',(#554),#39,.T.);
#4779=ADVANCED_FACE('',(#555),#4527,.T.);
#4780=ADVANCED_FACE('',(#556),#40,.T.);
#4781=ADVANCED_FACE('',(#557),#312,.F.);
#4782=ADVANCED_FACE('',(#558),#4528,.T.);
#4783=ADVANCED_FACE('',(#559,#104),#313,.F.);
#4784=ADVANCED_FACE('',(#560),#4529,.T.);
#4785=ADVANCED_FACE('',(#561),#314,.F.);
#4786=ADVANCED_FACE('',(#562),#51,.T.);
#4787=ADVANCED_FACE('',(#563),#4530,.T.);
#4788=ADVANCED_FACE('',(#564),#52,.T.);
#4789=ADVANCED_FACE('',(#565),#61,.F.);
#4790=ADVANCED_FACE('',(#566),#4531,.F.);
#4791=ADVANCED_FACE('',(#567),#4532,.T.);
#4792=ADVANCED_FACE('',(#568),#315,.F.);
#4793=ADVANCED_FACE('',(#569),#4533,.T.);
#4794=ADVANCED_FACE('',(#570),#4534,.F.);
#4795=ADVANCED_FACE('',(#571),#4535,.T.);
#4796=ADVANCED_FACE('',(#572),#4536,.T.);
#4797=ADVANCED_FACE('',(#573),#4537,.T.);
#4798=ADVANCED_FACE('',(#574),#53,.T.);
#4799=ADVANCED_FACE('',(#575),#41,.T.);
#4800=ADVANCED_FACE('',(#576),#4538,.T.);
#4801=ADVANCED_FACE('',(#577),#42,.T.);
#4802=ADVANCED_FACE('',(#578),#316,.T.);
#4803=ADVANCED_FACE('',(#579),#4539,.T.);
#4804=ADVANCED_FACE('',(#580,#105),#317,.T.);
#4805=ADVANCED_FACE('',(#581),#4540,.T.);
#4806=ADVANCED_FACE('',(#582),#318,.T.);
#4807=ADVANCED_FACE('',(#583),#54,.T.);
#4808=ADVANCED_FACE('',(#584),#4541,.T.);
#4809=ADVANCED_FACE('',(#585),#55,.T.);
#4810=ADVANCED_FACE('',(#586),#62,.F.);
#4811=ADVANCED_FACE('',(#587),#4542,.F.);
#4812=ADVANCED_FACE('',(#588),#4543,.T.);
#4813=ADVANCED_FACE('',(#589),#319,.T.);
#4814=ADVANCED_FACE('',(#590),#4544,.T.);
#4815=ADVANCED_FACE('',(#591),#4545,.F.);
#4816=ADVANCED_FACE('',(#592),#4546,.F.);
#4817=ADVANCED_FACE('',(#593),#320,.T.);
#4818=ADVANCED_FACE('',(#594,#106,#107),#321,.T.);
#4819=ADVANCED_FACE('',(#595,#108),#322,.T.);
#4820=ADVANCED_FACE('',(#596),#4547,.T.);
#4821=ADVANCED_FACE('',(#597,#109),#323,.T.);
#4822=ADVANCED_FACE('',(#598),#4548,.T.);
#4823=ADVANCED_FACE('',(#599,#110),#324,.T.);
#4830=CLOSED_SHELL('',(#4776,#4777,#4778,#4779,#4780,#4781,#4782,#4783,
#4784,#4785,#4786,#4787,#4788,#4789,#4790,#4791,#4792,#4793,#4794,#4795,
#4796,#4797,#4798,#4799,#4800,#4801,#4802,#4803,#4804,#4805,#4806,#4807,
#4808,#4809,#4810,#4811,#4812,#4813,#4814,#4815,#4816,#4817,#4818,#4819,
#4820,#4821,#4822,#4823));
#5309=AXIS2_PLACEMENT_3D('',#19629,#6532,#6533);
#5310=AXIS2_PLACEMENT_3D('',#19630,#6534,#6535);
#5311=AXIS2_PLACEMENT_3D('',#19633,#6536,#6537);
#5312=AXIS2_PLACEMENT_3D('',#19637,#6539,#6540);
#5313=AXIS2_PLACEMENT_3D('',#19639,#6542,#6543);
#5314=AXIS2_PLACEMENT_3D('',#19642,#6544,#6545);
#5315=AXIS2_PLACEMENT_3D('',#19643,#6546,#6547);
#5316=AXIS2_PLACEMENT_3D('',#19645,#6548,#6549);
#5317=AXIS2_PLACEMENT_3D('',#19646,#6550,#6551);
#5318=AXIS2_PLACEMENT_3D('',#19647,#6552,#6553);
#5319=AXIS2_PLACEMENT_3D('',#19648,#6554,#6555);
#5320=AXIS2_PLACEMENT_3D('',#19649,#6556,#6557);
#5321=AXIS2_PLACEMENT_3D('',#19651,#6558,#6559);
#5322=AXIS2_PLACEMENT_3D('',#19655,#6561,#6562);
#5323=AXIS2_PLACEMENT_3D('',#19657,#6564,#6565);
#5324=AXIS2_PLACEMENT_3D('',#19658,#6566,#6567);
#5325=AXIS2_PLACEMENT_3D('',#19659,#6568,#6569);
#5326=AXIS2_PLACEMENT_3D('',#19669,#6575,#6576);
#5327=AXIS2_PLACEMENT_3D('',#19671,#6577,#6578);
#5328=AXIS2_PLACEMENT_3D('',#19673,#6580,#6581);
#5329=AXIS2_PLACEMENT_3D('',#19675,#6582,#6583);
#5330=AXIS2_PLACEMENT_3D('',#19679,#6585,#6586);
#5331=AXIS2_PLACEMENT_3D('',#19682,#6588,#6589);
#5332=AXIS2_PLACEMENT_3D('',#19683,#6590,#6591);
#5333=AXIS2_PLACEMENT_3D('',#19685,#6592,#6593);
#5334=AXIS2_PLACEMENT_3D('',#19687,#6595,#6596);
#5335=AXIS2_PLACEMENT_3D('',#19695,#6601,#6602);
#5336=AXIS2_PLACEMENT_3D('',#19697,#6603,#6604);
#5337=AXIS2_PLACEMENT_3D('',#19698,#6605,#6606);
#5338=AXIS2_PLACEMENT_3D('',#19699,#6607,#6608);
#5339=AXIS2_PLACEMENT_3D('',#19701,#6609,#6610);
#5340=AXIS2_PLACEMENT_3D('',#19703,#6612,#6613);
#5341=AXIS2_PLACEMENT_3D('',#19704,#6614,#6615);
#5342=AXIS2_PLACEMENT_3D('',#19705,#6616,#6617);
#5343=AXIS2_PLACEMENT_3D('',#19707,#6618,#6619);
#5344=AXIS2_PLACEMENT_3D('',#19709,#6621,#6622);
#5345=AXIS2_PLACEMENT_3D('',#19711,#6623,#6624);
#5346=AXIS2_PLACEMENT_3D('',#19713,#6626,#6627);
#5347=AXIS2_PLACEMENT_3D('',#19715,#6628,#6629);
#5348=AXIS2_PLACEMENT_3D('',#19717,#6631,#6632);
#5349=AXIS2_PLACEMENT_3D('',#19721,#6635,#6636);
#5350=AXIS2_PLACEMENT_3D('',#19722,#6637,#6638);
#5351=AXIS2_PLACEMENT_3D('',#19723,#6639,#6640);
#5352=AXIS2_PLACEMENT_3D('',#19724,#6641,#6642);
#5353=AXIS2_PLACEMENT_3D('',#19725,#6643,#6644);
#5354=AXIS2_PLACEMENT_3D('',#19727,#6645,#6646);
#5355=AXIS2_PLACEMENT_3D('',#19730,#6648,#6649);
#5356=AXIS2_PLACEMENT_3D('',#19731,#6650,#6651);
#5357=AXIS2_PLACEMENT_3D('',#19733,#6652,#6653);
#5358=AXIS2_PLACEMENT_3D('',#19736,#6655,#6656);
#5359=AXIS2_PLACEMENT_3D('',#19737,#6657,#6658);
#5360=AXIS2_PLACEMENT_3D('',#19740,#6659,#6660);
#5361=AXIS2_PLACEMENT_3D('',#19744,#6662,#6663);
#5362=AXIS2_PLACEMENT_3D('',#19746,#6665,#6666);
#5363=AXIS2_PLACEMENT_3D('',#19749,#6667,#6668);
#5364=AXIS2_PLACEMENT_3D('',#19751,#6669,#6670);
#5365=AXIS2_PLACEMENT_3D('',#19752,#6671,#6672);
#5366=AXIS2_PLACEMENT_3D('',#19753,#6673,#6674);
#5367=AXIS2_PLACEMENT_3D('',#19754,#6675,#6676);
#5368=AXIS2_PLACEMENT_3D('',#19755,#6677,#6678);
#5369=AXIS2_PLACEMENT_3D('',#19756,#6679,#6680);
#5370=AXIS2_PLACEMENT_3D('',#19758,#6681,#6682);
#5371=AXIS2_PLACEMENT_3D('',#19762,#6684,#6685);
#5372=AXIS2_PLACEMENT_3D('',#19764,#6687,#6688);
#5373=AXIS2_PLACEMENT_3D('',#19765,#6689,#6690);
#5374=AXIS2_PLACEMENT_3D('',#19766,#6691,#6692);
#5375=AXIS2_PLACEMENT_3D('',#19773,#6697,#6698);
#5376=AXIS2_PLACEMENT_3D('',#19776,#6700,#6701);
#5377=AXIS2_PLACEMENT_3D('',#19777,#6702,#6703);
#5378=AXIS2_PLACEMENT_3D('',#19781,#6705,#6706);
#5379=AXIS2_PLACEMENT_3D('',#19784,#6708,#6709);
#5380=AXIS2_PLACEMENT_3D('',#19786,#6710,#6711);
#5381=AXIS2_PLACEMENT_3D('',#19787,#6712,#6713);
#5382=AXIS2_PLACEMENT_3D('',#19790,#6715,#6716);
#5383=AXIS2_PLACEMENT_3D('',#19791,#6717,#6718);
#5384=AXIS2_PLACEMENT_3D('',#19796,#6722,#6723);
#5385=AXIS2_PLACEMENT_3D('',#19798,#6724,#6725);
#5386=AXIS2_PLACEMENT_3D('',#19799,#6726,#6727);
#5387=AXIS2_PLACEMENT_3D('',#19800,#6728,#6729);
#5388=AXIS2_PLACEMENT_3D('',#19802,#6730,#6731);
#5389=AXIS2_PLACEMENT_3D('',#19804,#6733,#6734);
#5390=AXIS2_PLACEMENT_3D('',#19805,#6735,#6736);
#5391=AXIS2_PLACEMENT_3D('',#19806,#6737,#6738);
#5392=AXIS2_PLACEMENT_3D('',#19808,#6739,#6740);
#5393=AXIS2_PLACEMENT_3D('',#19810,#6742,#6743);
#5394=AXIS2_PLACEMENT_3D('',#19813,#6745,#6746);
#5395=AXIS2_PLACEMENT_3D('',#19814,#6747,#6748);
#5396=AXIS2_PLACEMENT_3D('',#19817,#6750,#6751);
#5397=AXIS2_PLACEMENT_3D('',#19818,#6752,#6753);
#5398=AXIS2_PLACEMENT_3D('',#19822,#6756,#6757);
#5399=AXIS2_PLACEMENT_3D('',#19823,#6758,#6759);
#5400=AXIS2_PLACEMENT_3D('',#19824,#6760,#6761);
#5401=AXIS2_PLACEMENT_3D('',#19825,#6762,#6763);
#5402=AXIS2_PLACEMENT_3D('',#19826,#6764,#6765);
#5403=AXIS2_PLACEMENT_3D('',#19828,#6766,#6767);
#5404=AXIS2_PLACEMENT_3D('',#19831,#6769,#6770);
#5405=AXIS2_PLACEMENT_3D('',#19832,#6771,#6772);
#5406=AXIS2_PLACEMENT_3D('',#19833,#6773,#6774);
#5407=AXIS2_PLACEMENT_3D('',#19834,#6775,#6776);
#5408=AXIS2_PLACEMENT_3D('',#19836,#6777,#6778);
#5409=AXIS2_PLACEMENT_3D('',#19837,#6779,#6780);
#5410=AXIS2_PLACEMENT_3D('',#19839,#6781,#6782);
#5411=AXIS2_PLACEMENT_3D('',#19841,#6784,#6785);
#5412=AXIS2_PLACEMENT_3D('',#19843,#6786,#6787);
#5413=AXIS2_PLACEMENT_3D('',#19844,#6788,#6789);
#5414=AXIS2_PLACEMENT_3D('',#19846,#6790,#6791);
#5415=AXIS2_PLACEMENT_3D('',#19848,#6793,#6794);
#6532=DIRECTION('axis',(0.,0.,1.));
#6533=DIRECTION('refdir',(1.,0.,0.));
#6534=DIRECTION('center_axis',(0.,0.,1.));
#6535=DIRECTION('ref_axis',(-0.894892375881552,-0.446282013517317,0.));
#6536=DIRECTION('center_axis',(0.,0.,1.));
#6537=DIRECTION('ref_axis',(-0.79874874277943,0.601664728821858,0.));
#6538=DIRECTION('',(0.,0.,1.));
#6539=DIRECTION('center_axis',(0.,0.,1.));
#6540=DIRECTION('ref_axis',(-0.894892375881552,-0.446282013517317,0.));
#6541=DIRECTION('',(0.,0.,-1.));
#6542=DIRECTION('center_axis',(0.,0.,1.));
#6543=DIRECTION('ref_axis',(1.,-1.22464679914735E-16,0.));
#6544=DIRECTION('center_axis',(-0.601664728821861,0.798748742779428,-3.54715698049647E-15));
#6545=DIRECTION('ref_axis',(-0.798748742779428,-0.601664728821861,-1.85390118736899E-31));
#6546=DIRECTION('center_axis',(0.,0.,1.));
#6547=DIRECTION('ref_axis',(1.,1.22464679914735E-16,0.));
#6548=DIRECTION('center_axis',(-0.601664728821861,-0.798748742779428,-3.54715698049647E-15));
#6549=DIRECTION('ref_axis',(2.50378775993336E-30,-4.44089209850063E-15,
1.));
#6550=DIRECTION('center_axis',(0.,0.,-1.));
#6551=DIRECTION('ref_axis',(1.,1.22464679914735E-16,0.));
#6552=DIRECTION('center_axis',(0.185467508428577,-0.954822547310801,-0.232197559126295));
#6553=DIRECTION('ref_axis',(-0.595903538017452,-0.297176552148574,0.746046292284446));
#6554=DIRECTION('center_axis',(1.,0.,0.));
#6555=DIRECTION('ref_axis',(0.,-0.707106781186546,0.707106781186549));
#6556=DIRECTION('center_axis',(0.,0.,1.));
#6557=DIRECTION('ref_axis',(-0.894892375881552,0.446282013517317,0.));
#6558=DIRECTION('center_axis',(0.,0.,1.));
#6559=DIRECTION('ref_axis',(0.,1.,0.));
#6560=DIRECTION('',(0.,0.,1.));
#6561=DIRECTION('center_axis',(0.,0.,1.));
#6562=DIRECTION('ref_axis',(-0.894892375881552,0.446282013517317,0.));
#6563=DIRECTION('',(0.,0.,-1.));
#6564=DIRECTION('center_axis',(-0.185467508428577,-0.954822547310802,0.23219755912629));
#6565=DIRECTION('ref_axis',(-0.595903538017456,0.297176552148567,0.746046292284445));
#6566=DIRECTION('center_axis',(1.,0.,0.));
#6567=DIRECTION('ref_axis',(0.,0.707106781186546,0.707106781186549));
#6568=DIRECTION('center_axis',(0.,1.,0.));
#6569=DIRECTION('ref_axis',(1.,0.,0.));
#6570=DIRECTION('',(1.,0.,0.));
#6571=DIRECTION('',(0.,0.,1.));
#6572=DIRECTION('',(1.,0.,0.));
#6573=DIRECTION('',(0.,0.,1.));
#6574=DIRECTION('',(-1.,0.,0.));
#6575=DIRECTION('center_axis',(-1.,0.,0.));
#6576=DIRECTION('ref_axis',(0.,-0.707106781186547,0.707106781186548));
#6577=DIRECTION('center_axis',(1.,0.,0.));
#6578=DIRECTION('ref_axis',(0.,0.,1.));
#6579=DIRECTION('',(1.,0.,0.));
#6580=DIRECTION('center_axis',(0.,0.,-1.));
#6581=DIRECTION('ref_axis',(-1.,0.,0.));
#6582=DIRECTION('center_axis',(0.,0.,1.));
#6583=DIRECTION('ref_axis',(0.707106781186548,-0.707106781186547,0.));
#6584=DIRECTION('',(0.,1.,0.));
#6585=DIRECTION('center_axis',(0.,0.,1.));
#6586=DIRECTION('ref_axis',(0.707106781186548,0.707106781186547,0.));
#6587=DIRECTION('',(-1.,0.,0.));
#6588=DIRECTION('center_axis',(0.,0.,-1.));
#6589=DIRECTION('ref_axis',(-1.,0.,0.));
#6590=DIRECTION('center_axis',(1.,0.,0.));
#6591=DIRECTION('ref_axis',(0.,0.707106781186547,0.707106781186548));
#6592=DIRECTION('center_axis',(-1.,0.,0.));
#6593=DIRECTION('ref_axis',(0.,0.,1.));
#6594=DIRECTION('',(1.,0.,0.));
#6595=DIRECTION('center_axis',(0.,-1.,0.));
#6596=DIRECTION('ref_axis',(-1.,0.,0.));
#6597=DIRECTION('',(0.,0.,-1.));
#6598=DIRECTION('',(-1.,0.,0.));
#6599=DIRECTION('',(0.,0.,-1.));
#6600=DIRECTION('',(-1.,0.,0.));
#6601=DIRECTION('center_axis',(0.,0.,-1.));
#6602=DIRECTION('ref_axis',(1.,0.,0.));
#6603=DIRECTION('center_axis',(2.22044604925032E-15,1.,0.));
#6604=DIRECTION('ref_axis',(0.,0.,1.));
#6605=DIRECTION('center_axis',(0.,0.,-1.));
#6606=DIRECTION('ref_axis',(0.707106781186548,-0.707106781186547,0.));
#6607=DIRECTION('center_axis',(0.,-1.,0.));
#6608=DIRECTION('ref_axis',(0.707106781186547,0.,0.707106781186548));
#6609=DIRECTION('center_axis',(-2.22044604925032E-15,1.,0.));
#6610=DIRECTION('ref_axis',(0.,0.,1.));
#6611=DIRECTION('',(0.,-1.,0.));
#6612=DIRECTION('center_axis',(0.,0.,-1.));
#6613=DIRECTION('ref_axis',(1.,0.,0.));
#6614=DIRECTION('center_axis',(0.,0.,-1.));
#6615=DIRECTION('ref_axis',(0.707106781186548,0.707106781186547,0.));
#6616=DIRECTION('center_axis',(0.,0.,1.));
#6617=DIRECTION('ref_axis',(-1.,0.,0.));
#6618=DIRECTION('center_axis',(0.,0.,1.));
#6619=DIRECTION('ref_axis',(-1.,0.,0.));
#6620=DIRECTION('',(0.707106781186548,8.65956056235494E-17,0.707106781186547));
#6621=DIRECTION('center_axis',(0.,0.,1.));
#6622=DIRECTION('ref_axis',(-1.,0.,0.));
#6623=DIRECTION('center_axis',(0.,0.,-1.));
#6624=DIRECTION('ref_axis',(-1.,0.,0.));
#6625=DIRECTION('',(0.,0.,1.));
#6626=DIRECTION('center_axis',(0.,0.,1.));
#6627=DIRECTION('ref_axis',(0.707106781186548,-0.707106781186548,0.));
#6628=DIRECTION('center_axis',(0.,0.,-1.));
#6629=DIRECTION('ref_axis',(0.707106781186548,-0.707106781186548,0.));
#6630=DIRECTION('',(0.,0.,-1.));
#6631=DIRECTION('center_axis',(-1.,0.,0.));
#6632=DIRECTION('ref_axis',(0.,1.,0.));
#6633=DIRECTION('',(0.,1.,0.));
#6634=DIRECTION('',(0.,0.,1.));
#6635=DIRECTION('center_axis',(0.,0.,1.));
#6636=DIRECTION('ref_axis',(0.707106781186548,0.707106781186548,0.));
#6637=DIRECTION('center_axis',(0.,0.,-1.));
#6638=DIRECTION('ref_axis',(0.707106781186548,0.707106781186548,0.));
#6639=DIRECTION('center_axis',(0.,0.,1.));
#6640=DIRECTION('ref_axis',(1.,-1.22464679914735E-16,0.));
#6641=DIRECTION('center_axis',(0.,0.,1.));
#6642=DIRECTION('ref_axis',(-1.,0.,0.));
#6643=DIRECTION('center_axis',(0.,0.,1.));
#6644=DIRECTION('ref_axis',(1.,0.,0.));
#6645=DIRECTION('center_axis',(0.,0.,-1.));
#6646=DIRECTION('ref_axis',(1.,0.,0.));
#6647=DIRECTION('',(0.,0.,1.));
#6648=DIRECTION('center_axis',(0.,0.,1.));
#6649=DIRECTION('ref_axis',(1.,0.,0.));
#6650=DIRECTION('center_axis',(0.,0.,1.));
#6651=DIRECTION('ref_axis',(1.,0.,0.));
#6652=DIRECTION('center_axis',(0.,0.,1.));
#6653=DIRECTION('ref_axis',(1.,0.,0.));
#6654=DIRECTION('',(0.,0.,-1.));
#6655=DIRECTION('center_axis',(0.,0.,-1.));
#6656=DIRECTION('ref_axis',(1.,0.,0.));
#6657=DIRECTION('center_axis',(0.,0.,-1.));
#6658=DIRECTION('ref_axis',(0.894892375881552,-0.446282013517317,0.));
#6659=DIRECTION('center_axis',(0.,0.,-1.));
#6660=DIRECTION('ref_axis',(0.79874874277943,0.601664728821858,0.));
#6661=DIRECTION('',(0.,0.,-1.));
#6662=DIRECTION('center_axis',(0.,0.,-1.));
#6663=DIRECTION('ref_axis',(0.894892375881552,-0.446282013517317,0.));
#6664=DIRECTION('',(0.,0.,1.));
#6665=DIRECTION('center_axis',(0.,0.,1.));
#6666=DIRECTION('ref_axis',(-1.,1.22464679914735E-16,0.));
#6667=DIRECTION('center_axis',(-0.601664728821861,-0.798748742779428,3.54715698049647E-15));
#6668=DIRECTION('ref_axis',(0.798748742779428,-0.601664728821861,-1.85390118736899E-31));
#6669=DIRECTION('center_axis',(0.,0.,1.));
#6670=DIRECTION('ref_axis',(-1.,1.22464679914735E-16,0.));
#6671=DIRECTION('center_axis',(-0.601664728821861,0.798748742779428,3.54715698049647E-15));
#6672=DIRECTION('ref_axis',(-2.50378775993336E-30,-4.44089209850063E-15,
1.));
#6673=DIRECTION('center_axis',(0.,0.,-1.));
#6674=DIRECTION('ref_axis',(-1.,1.22464679914735E-16,0.));
#6675=DIRECTION('center_axis',(-0.185467508428577,-0.954822547310801,-0.232197559126295));
#6676=DIRECTION('ref_axis',(0.595903538017452,-0.297176552148574,0.746046292284446));
#6677=DIRECTION('center_axis',(1.,0.,0.));
#6678=DIRECTION('ref_axis',(0.,-0.707106781186546,0.707106781186549));
#6679=DIRECTION('center_axis',(0.,0.,-1.));
#6680=DIRECTION('ref_axis',(0.894892375881552,0.446282013517317,0.));
#6681=DIRECTION('center_axis',(0.,0.,-1.));
#6682=DIRECTION('ref_axis',(0.,1.,0.));
#6683=DIRECTION('',(0.,0.,-1.));
#6684=DIRECTION('center_axis',(0.,0.,-1.));
#6685=DIRECTION('ref_axis',(0.894892375881552,0.446282013517317,0.));
#6686=DIRECTION('',(0.,0.,1.));
#6687=DIRECTION('center_axis',(0.185467508428577,-0.954822547310802,0.23219755912629));
#6688=DIRECTION('ref_axis',(0.595903538017456,0.297176552148567,0.746046292284445));
#6689=DIRECTION('center_axis',(1.,0.,0.));
#6690=DIRECTION('ref_axis',(0.,0.707106781186546,0.707106781186549));
#6691=DIRECTION('center_axis',(0.,-1.,0.));
#6692=DIRECTION('ref_axis',(-1.,0.,0.));
#6693=DIRECTION('',(-1.,0.,0.));
#6694=DIRECTION('',(1.,0.,0.));
#6695=DIRECTION('',(0.,0.,1.));
#6696=DIRECTION('',(-1.,0.,0.));
#6697=DIRECTION('center_axis',(-1.,0.,0.));
#6698=DIRECTION('ref_axis',(0.,-0.707106781186547,0.707106781186548));
#6699=DIRECTION('',(-1.,0.,0.));
#6700=DIRECTION('center_axis',(1.,0.,0.));
#6701=DIRECTION('ref_axis',(0.,0.,1.));
#6702=DIRECTION('center_axis',(0.,0.,1.));
#6703=DIRECTION('ref_axis',(1.,0.,0.));
#6704=DIRECTION('',(1.,0.,0.));
#6705=DIRECTION('center_axis',(0.,0.,-1.));
#6706=DIRECTION('ref_axis',(-0.707106781186548,0.707106781186547,0.));
#6707=DIRECTION('',(0.,1.,0.));
#6708=DIRECTION('center_axis',(0.,0.,-1.));
#6709=DIRECTION('ref_axis',(-0.707106781186548,-0.707106781186547,0.));
#6710=DIRECTION('center_axis',(0.,0.,1.));
#6711=DIRECTION('ref_axis',(1.,0.,0.));
#6712=DIRECTION('center_axis',(1.,0.,0.));
#6713=DIRECTION('ref_axis',(0.,0.707106781186547,0.707106781186548));
#6714=DIRECTION('',(-1.,0.,0.));
#6715=DIRECTION('center_axis',(-1.,0.,0.));
#6716=DIRECTION('ref_axis',(0.,0.,1.));
#6717=DIRECTION('center_axis',(0.,1.,0.));
#6718=DIRECTION('ref_axis',(1.,0.,0.));
#6719=DIRECTION('',(1.,0.,0.));
#6720=DIRECTION('',(1.,0.,0.));
#6721=DIRECTION('',(0.,0.,-1.));
#6722=DIRECTION('center_axis',(0.,0.,-1.));
#6723=DIRECTION('ref_axis',(-1.,0.,0.));
#6724=DIRECTION('center_axis',(2.22044604925032E-15,-1.,0.));
#6725=DIRECTION('ref_axis',(0.,0.,1.));
#6726=DIRECTION('center_axis',(0.,0.,1.));
#6727=DIRECTION('ref_axis',(-0.707106781186548,-0.707106781186547,0.));
#6728=DIRECTION('center_axis',(0.,1.,0.));
#6729=DIRECTION('ref_axis',(-0.707106781186547,0.,0.707106781186548));
#6730=DIRECTION('center_axis',(-2.22044604925032E-15,-1.,0.));
#6731=DIRECTION('ref_axis',(0.,0.,1.));
#6732=DIRECTION('',(0.,-1.,0.));
#6733=DIRECTION('center_axis',(0.,0.,-1.));
#6734=DIRECTION('ref_axis',(-1.,0.,0.));
#6735=DIRECTION('center_axis',(0.,0.,1.));
#6736=DIRECTION('ref_axis',(-0.707106781186548,0.707106781186547,0.));
#6737=DIRECTION('center_axis',(0.,0.,1.));
#6738=DIRECTION('ref_axis',(1.,0.,0.));
#6739=DIRECTION('center_axis',(0.,0.,-1.));
#6740=DIRECTION('ref_axis',(1.,0.,0.));
#6741=DIRECTION('',(-0.707106781186548,-8.65956056235494E-17,0.707106781186547));
#6742=DIRECTION('center_axis',(0.,0.,-1.));
#6743=DIRECTION('ref_axis',(1.,0.,0.));
#6744=DIRECTION('',(0.,0.,-1.));
#6745=DIRECTION('center_axis',(0.,0.,1.));
#6746=DIRECTION('ref_axis',(1.,0.,0.));
#6747=DIRECTION('center_axis',(0.,0.,-1.));
#6748=DIRECTION('ref_axis',(-0.707106781186548,-0.707106781186548,0.));
#6749=DIRECTION('',(0.,0.,-1.));
#6750=DIRECTION('center_axis',(0.,0.,1.));
#6751=DIRECTION('ref_axis',(-0.707106781186548,-0.707106781186548,0.));
#6752=DIRECTION('center_axis',(-1.,0.,0.));
#6753=DIRECTION('ref_axis',(0.,1.,0.));
#6754=DIRECTION('',(0.,0.,1.));
#6755=DIRECTION('',(0.,1.,0.));
#6756=DIRECTION('center_axis',(0.,0.,-1.));
#6757=DIRECTION('ref_axis',(-0.707106781186548,0.707106781186548,0.));
#6758=DIRECTION('center_axis',(0.,0.,1.));
#6759=DIRECTION('ref_axis',(-0.707106781186548,0.707106781186548,0.));
#6760=DIRECTION('center_axis',(0.,0.,-1.));
#6761=DIRECTION('ref_axis',(-1.,-1.22464679914735E-16,0.));
#6762=DIRECTION('center_axis',(0.,0.,-1.));
#6763=DIRECTION('ref_axis',(1.,0.,0.));
#6764=DIRECTION('center_axis',(0.,0.,1.));
#6765=DIRECTION('ref_axis',(1.,0.,0.));
#6766=DIRECTION('center_axis',(0.,0.,1.));
#6767=DIRECTION('ref_axis',(1.,0.,0.));
#6768=DIRECTION('',(0.,0.,1.));
#6769=DIRECTION('center_axis',(0.,0.,1.));
#6770=DIRECTION('ref_axis',(1.,0.,0.));
#6771=DIRECTION('center_axis',(0.,0.,1.));
#6772=DIRECTION('ref_axis',(1.,0.,0.));
#6773=DIRECTION('center_axis',(0.,0.,-1.));
#6774=DIRECTION('ref_axis',(-1.,0.,0.));
#6775=DIRECTION('center_axis',(0.,0.,1.));
#6776=DIRECTION('ref_axis',(1.,0.,0.));
#6777=DIRECTION('center_axis',(0.,0.,1.));
#6778=DIRECTION('ref_axis',(1.,0.,0.));
#6779=DIRECTION('center_axis',(0.,0.,1.));
#6780=DIRECTION('ref_axis',(1.,0.,0.));
#6781=DIRECTION('center_axis',(0.,0.,1.));
#6782=DIRECTION('ref_axis',(1.,0.,0.));
#6783=DIRECTION('',(0.,0.,-1.));
#6784=DIRECTION('center_axis',(0.,0.,1.));
#6785=DIRECTION('ref_axis',(1.,0.,0.));
#6786=DIRECTION('center_axis',(0.,0.,1.));
#6787=DIRECTION('ref_axis',(1.,0.,0.));
#6788=DIRECTION('center_axis',(0.,0.,1.));
#6789=DIRECTION('ref_axis',(1.,0.,0.));
#6790=DIRECTION('center_axis',(0.,0.,1.));
#6791=DIRECTION('ref_axis',(1.,0.,0.));
#6792=DIRECTION('',(0.,0.,-1.));
#6793=DIRECTION('center_axis',(0.,0.,1.));
#6794=DIRECTION('ref_axis',(1.,0.,0.));
#19629=CARTESIAN_POINT('',(0.,0.,0.));
#19630=CARTESIAN_POINT('Origin',(31.8615483148624,-24.,0.));
#19631=CARTESIAN_POINT('',(31.062799572083,-23.3983352711781,-6.));
#19632=CARTESIAN_POINT('',(31.8615483148624,-25.,-6.));
#19633=CARTESIAN_POINT('Origin',(31.8615483148624,-24.,-6.));
#19634=CARTESIAN_POINT('',(31.062799572083,-23.3983352711781,-10.));
#19635=CARTESIAN_POINT('',(31.062799572083,-23.3983352711781,0.));
#19636=CARTESIAN_POINT('',(31.8615483148624,-25.,-10.));
#19637=CARTESIAN_POINT('Origin',(31.8615483148624,-24.,-10.));
#19638=CARTESIAN_POINT('',(31.8615483148624,-25.,0.));
#19639=CARTESIAN_POINT('Origin',(0.,0.,-6.));
#19640=CARTESIAN_POINT('',(31.062799572083,23.3983352711781,-6.));
#19641=CARTESIAN_POINT('',(31.8615483148624,24.,-5.));
#19642=CARTESIAN_POINT('Origin',(31.8615483148624,24.,-6.));
#19643=CARTESIAN_POINT('Origin',(0.,0.,-6.));
#19644=CARTESIAN_POINT('',(31.8615483148624,-24.,-5.));
#19645=CARTESIAN_POINT('Origin',(31.8615483148624,-24.,-6.));
#19646=CARTESIAN_POINT('Origin',(0.,0.,-5.));
#19647=CARTESIAN_POINT('Origin',(31.8615483148624,-24.,-6.));
#19648=CARTESIAN_POINT('Origin',(31.8615483148624,-24.,-6.));
#19649=CARTESIAN_POINT('Origin',(31.8615483148624,24.,0.));
#19650=CARTESIAN_POINT('',(31.8615483148624,25.,-6.));
#19651=CARTESIAN_POINT('Origin',(31.8615483148624,24.,-6.));
#19652=CARTESIAN_POINT('',(31.8615483148624,25.,-10.));
#19653=CARTESIAN_POINT('',(31.8615483148624,25.,0.));
#19654=CARTESIAN_POINT('',(31.062799572083,23.3983352711781,-10.));
#19655=CARTESIAN_POINT('Origin',(31.8615483148624,24.,-10.));
#19656=CARTESIAN_POINT('',(31.062799572083,23.3983352711781,0.));
#19657=CARTESIAN_POINT('Origin',(31.8615483148624,24.,-6.));
#19658=CARTESIAN_POINT('Origin',(31.8615483148624,24.,-6.));
#19659=CARTESIAN_POINT('Origin',(29.7889175821791,-25.,0.));
#19660=CARTESIAN_POINT('',(21.540659228538,-25.,-10.));
#19661=CARTESIAN_POINT('',(25.8778257092103,-25.,-10.));
#19662=CARTESIAN_POINT('',(21.540659228538,-25.,-14.));
#19663=CARTESIAN_POINT('',(21.540659228538,-25.,-11.));
#19664=CARTESIAN_POINT('',(70.,-25.,-14.));
#19665=CARTESIAN_POINT('',(75.,-25.,-14.));
#19666=CARTESIAN_POINT('',(70.,-25.,-6.));
#19667=CARTESIAN_POINT('',(70.,-25.,0.));
#19668=CARTESIAN_POINT('',(41.0916881866343,-25.,-6.));
#19669=CARTESIAN_POINT('Origin',(41.0916881866343,-24.,-6.));
#19670=CARTESIAN_POINT('',(70.,-24.,-5.));
#19671=CARTESIAN_POINT('Origin',(70.,-24.,-6.));
#19672=CARTESIAN_POINT('',(41.0916881866343,-24.,-5.));
#19673=CARTESIAN_POINT('Origin',(52.3944587910896,0.,-5.));
#19674=CARTESIAN_POINT('',(74.,-20.,-5.));
#19675=CARTESIAN_POINT('Origin',(70.,-20.,-5.));
#19676=CARTESIAN_POINT('',(74.,20.,-5.));
#19677=CARTESIAN_POINT('',(74.,-12.5,-5.));
#19678=CARTESIAN_POINT('',(70.,24.,-5.));
#19679=CARTESIAN_POINT('Origin',(70.,20.,-5.));
#19680=CARTESIAN_POINT('',(63.6972293955448,24.,-5.));
#19681=CARTESIAN_POINT('',(71.5444185458617,-1.3259677713873E-15,-5.));
#19682=CARTESIAN_POINT('Origin',(60.7170700212872,0.,-5.));
#19683=CARTESIAN_POINT('Origin',(63.6972293955448,24.,-6.));
#19684=CARTESIAN_POINT('',(70.,25.,-6.));
#19685=CARTESIAN_POINT('Origin',(70.,24.,-6.));
#19686=CARTESIAN_POINT('',(63.6972293955448,25.,-6.));
#19687=CARTESIAN_POINT('Origin',(75.,25.,0.));
#19688=CARTESIAN_POINT('',(70.,25.,-14.));
#19689=CARTESIAN_POINT('',(70.,25.,0.));
#19690=CARTESIAN_POINT('',(21.540659228538,25.,-14.));
#19691=CARTESIAN_POINT('',(-75.,25.,-14.));
#19692=CARTESIAN_POINT('',(21.540659228538,25.,-10.));
#19693=CARTESIAN_POINT('',(21.540659228538,25.,-11.));
#19694=CARTESIAN_POINT('',(30.0019548860308,25.,-10.));
#19695=CARTESIAN_POINT('Origin',(70.,-20.,-6.));
#19696=CARTESIAN_POINT('',(75.,-20.,-6.));
#19697=CARTESIAN_POINT('Origin',(74.,-20.,-6.));
#19698=CARTESIAN_POINT('Origin',(70.,-20.,-6.));
#19699=CARTESIAN_POINT('Origin',(74.,-12.5,-6.));
#19700=CARTESIAN_POINT('',(75.,20.,-6.));
#19701=CARTESIAN_POINT('Origin',(74.,20.,-6.));
#19702=CARTESIAN_POINT('',(75.,-12.5,-6.));
#19703=CARTESIAN_POINT('Origin',(70.,20.,-6.));
#19704=CARTESIAN_POINT('Origin',(70.,20.,-6.));
#19705=CARTESIAN_POINT('Origin',(60.7170700212872,0.,-6.));
#19706=CARTESIAN_POINT('',(69.5444185458617,1.08103841155783E-15,-7.));
#19707=CARTESIAN_POINT('Origin',(60.7170700212872,0.,-7.));
#19708=CARTESIAN_POINT('',(70.5444185458617,1.20350309147256E-15,-6.));
#19709=CARTESIAN_POINT('Origin',(60.7170700212872,0.,0.));
#19710=CARTESIAN_POINT('',(69.5444185458617,-1.08103841155783E-15,-14.));
#19711=CARTESIAN_POINT('Origin',(60.7170700212872,0.,-14.));
#19712=CARTESIAN_POINT('',(69.5444185458617,1.08103841155783E-15,0.));
#19713=CARTESIAN_POINT('Origin',(70.,-20.,0.));
#19714=CARTESIAN_POINT('',(75.,-20.,-14.));
#19715=CARTESIAN_POINT('Origin',(70.,-20.,-14.));
#19716=CARTESIAN_POINT('',(75.,-20.,0.));
#19717=CARTESIAN_POINT('Origin',(75.,-25.,0.));
#19718=CARTESIAN_POINT('',(75.,20.,-14.));
#19719=CARTESIAN_POINT('',(75.,25.,-14.));
#19720=CARTESIAN_POINT('',(75.,20.,0.));
#19721=CARTESIAN_POINT('Origin',(70.,20.,0.));
#19722=CARTESIAN_POINT('Origin',(70.,20.,-14.));
#19723=CARTESIAN_POINT('Origin',(0.,0.,0.));
#19724=CARTESIAN_POINT('Origin',(0.,0.,-10.));
#19725=CARTESIAN_POINT('Origin',(0.,0.,-11.));
#19726=CARTESIAN_POINT('',(-21.540659228538,25.,-14.));
#19727=CARTESIAN_POINT('Origin',(0.,0.,-14.));
#19728=CARTESIAN_POINT('',(-21.540659228538,25.,-10.));
#19729=CARTESIAN_POINT('',(-21.540659228538,25.,-11.));
#19730=CARTESIAN_POINT('Origin',(0.,0.,-10.));
#19731=CARTESIAN_POINT('Origin',(0.,0.,-11.));
#19732=CARTESIAN_POINT('',(-21.540659228538,-25.,-10.));
#19733=CARTESIAN_POINT('Origin',(0.,0.,-10.));
#19734=CARTESIAN_POINT('',(-21.540659228538,-25.,-14.));
#19735=CARTESIAN_POINT('',(-21.540659228538,-25.,-11.));
#19736=CARTESIAN_POINT('Origin',(0.,0.,-14.));
#19737=CARTESIAN_POINT('Origin',(-31.8615483148624,-24.,0.));
#19738=CARTESIAN_POINT('',(-31.062799572083,-23.3983352711781,-6.));
#19739=CARTESIAN_POINT('',(-31.8615483148624,-25.,-6.));
#19740=CARTESIAN_POINT('Origin',(-31.8615483148624,-24.,-6.));
#19741=CARTESIAN_POINT('',(-31.8615483148624,-25.,-10.));
#19742=CARTESIAN_POINT('',(-31.8615483148624,-25.,0.));
#19743=CARTESIAN_POINT('',(-31.062799572083,-23.3983352711781,-10.));
#19744=CARTESIAN_POINT('Origin',(-31.8615483148624,-24.,-10.));
#19745=CARTESIAN_POINT('',(-31.062799572083,-23.3983352711781,0.));
#19746=CARTESIAN_POINT('Origin',(0.,0.,-6.));
#19747=CARTESIAN_POINT('',(-31.062799572083,23.3983352711781,-6.));
#19748=CARTESIAN_POINT('',(-31.8615483148624,24.,-5.));
#19749=CARTESIAN_POINT('Origin',(-31.8615483148624,24.,-6.));
#19750=CARTESIAN_POINT('',(-31.8615483148624,-24.,-5.));
#19751=CARTESIAN_POINT('Origin',(0.,0.,-5.));
#19752=CARTESIAN_POINT('Origin',(-31.8615483148624,-24.,-6.));
#19753=CARTESIAN_POINT('Origin',(0.,0.,-6.));
#19754=CARTESIAN_POINT('Origin',(-31.8615483148624,-24.,-6.));
#19755=CARTESIAN_POINT('Origin',(-31.8615483148624,-24.,-6.));
#19756=CARTESIAN_POINT('Origin',(-31.8615483148624,24.,0.));
#19757=CARTESIAN_POINT('',(-31.8615483148624,25.,-6.));
#19758=CARTESIAN_POINT('Origin',(-31.8615483148624,24.,-6.));
#19759=CARTESIAN_POINT('',(-31.062799572083,23.3983352711781,-10.));
#19760=CARTESIAN_POINT('',(-31.062799572083,23.3983352711781,0.));
#19761=CARTESIAN_POINT('',(-31.8615483148624,25.,-10.));
#19762=CARTESIAN_POINT('Origin',(-31.8615483148624,24.,-10.));
#19763=CARTESIAN_POINT('',(-31.8615483148624,25.,0.));
#19764=CARTESIAN_POINT('Origin',(-31.8615483148624,24.,-6.));
#19765=CARTESIAN_POINT('Origin',(-31.8615483148624,24.,-6.));
#19766=CARTESIAN_POINT('Origin',(-29.7889175821791,-25.,0.));
#19767=CARTESIAN_POINT('',(-25.8778257092103,-25.,-10.));
#19768=CARTESIAN_POINT('',(-70.,-25.,-6.));
#19769=CARTESIAN_POINT('',(-41.0916881866343,-25.,-6.));
#19770=CARTESIAN_POINT('',(-70.,-25.,-14.));
#19771=CARTESIAN_POINT('',(-70.,-25.,0.));
#19772=CARTESIAN_POINT('',(-75.,-25.,-14.));
#19773=CARTESIAN_POINT('Origin',(-41.0916881866343,-24.,-6.));
#19774=CARTESIAN_POINT('',(-70.,-24.,-5.));
#19775=CARTESIAN_POINT('',(-41.0916881866343,-24.,-5.));
#19776=CARTESIAN_POINT('Origin',(-70.,-24.,-6.));
#19777=CARTESIAN_POINT('Origin',(-52.3944587910896,0.,-5.));
#19778=CARTESIAN_POINT('',(-70.,24.,-5.));
#19779=CARTESIAN_POINT('',(-63.6972293955448,24.,-5.));
#19780=CARTESIAN_POINT('',(-74.,20.,-5.));
#19781=CARTESIAN_POINT('Origin',(-70.,20.,-5.));
#19782=CARTESIAN_POINT('',(-74.,-20.,-5.));
#19783=CARTESIAN_POINT('',(-74.,-12.5,-5.));
#19784=CARTESIAN_POINT('Origin',(-70.,-20.,-5.));
#19785=CARTESIAN_POINT('',(-71.5444185458617,-1.3259677713873E-15,-5.));
#19786=CARTESIAN_POINT('Origin',(-60.7170700212872,0.,-5.));
#19787=CARTESIAN_POINT('Origin',(-63.6972293955448,24.,-6.));
#19788=CARTESIAN_POINT('',(-70.,25.,-6.));
#19789=CARTESIAN_POINT('',(-63.6972293955448,25.,-6.));
#19790=CARTESIAN_POINT('Origin',(-70.,24.,-6.));
#19791=CARTESIAN_POINT('Origin',(-75.,25.,0.));
#19792=CARTESIAN_POINT('',(-30.0019548860308,25.,-10.));
#19793=CARTESIAN_POINT('',(-70.,25.,-14.));
#19794=CARTESIAN_POINT('',(75.,25.,-14.));
#19795=CARTESIAN_POINT('',(-70.,25.,0.));
#19796=CARTESIAN_POINT('Origin',(-70.,-20.,-6.));
#19797=CARTESIAN_POINT('',(-75.,-20.,-6.));
#19798=CARTESIAN_POINT('Origin',(-74.,-20.,-6.));
#19799=CARTESIAN_POINT('Origin',(-70.,-20.,-6.));
#19800=CARTESIAN_POINT('Origin',(-74.,-12.5,-6.));
#19801=CARTESIAN_POINT('',(-75.,20.,-6.));
#19802=CARTESIAN_POINT('Origin',(-74.,20.,-6.));
#19803=CARTESIAN_POINT('',(-75.,-12.5,-6.));
#19804=CARTESIAN_POINT('Origin',(-70.,20.,-6.));
#19805=CARTESIAN_POINT('Origin',(-70.,20.,-6.));
#19806=CARTESIAN_POINT('Origin',(-60.7170700212872,0.,-6.));
#19807=CARTESIAN_POINT('',(-69.5444185458617,1.08103841155783E-15,-7.));
#19808=CARTESIAN_POINT('Origin',(-60.7170700212872,0.,-7.));
#19809=CARTESIAN_POINT('',(-70.5444185458617,-1.20350309147256E-15,-6.));
#19810=CARTESIAN_POINT('Origin',(-60.7170700212872,0.,0.));
#19811=CARTESIAN_POINT('',(-69.5444185458617,-1.08103841155783E-15,-14.));
#19812=CARTESIAN_POINT('',(-69.5444185458617,1.08103841155783E-15,0.));
#19813=CARTESIAN_POINT('Origin',(-60.7170700212872,0.,-14.));
#19814=CARTESIAN_POINT('Origin',(-70.,-20.,0.));
#19815=CARTESIAN_POINT('',(-75.,-20.,-14.));
#19816=CARTESIAN_POINT('',(-75.,-20.,0.));
#19817=CARTESIAN_POINT('Origin',(-70.,-20.,-14.));
#19818=CARTESIAN_POINT('Origin',(-75.,-25.,0.));
#19819=CARTESIAN_POINT('',(-75.,20.,-14.));
#19820=CARTESIAN_POINT('',(-75.,20.,0.));
#19821=CARTESIAN_POINT('',(-75.,25.,-14.));
#19822=CARTESIAN_POINT('Origin',(-70.,20.,0.));
#19823=CARTESIAN_POINT('Origin',(-70.,20.,-14.));
#19824=CARTESIAN_POINT('Origin',(0.,0.,0.));
#19825=CARTESIAN_POINT('Origin',(0.,0.,-10.));
#19826=CARTESIAN_POINT('Origin',(0.,0.,-7.83658590146904));
#19827=CARTESIAN_POINT('',(-27.4027293621977,-3.35586648013166E-15,-10.));
#19828=CARTESIAN_POINT('Origin',(0.,0.,-10.));
#19829=CARTESIAN_POINT('',(-27.4027293621977,-3.35586648013166E-15,-5.67317180293808));
#19830=CARTESIAN_POINT('',(-27.4027293621977,-3.35586648013166E-15,-7.83658590146904));
#19831=CARTESIAN_POINT('Origin',(0.,0.,-5.67317180293808));
#19832=CARTESIAN_POINT('Origin',(0.,0.,-10.));
#19833=CARTESIAN_POINT('Origin',(33.,0.,-14.));
#19834=CARTESIAN_POINT('Origin',(31.1192710879259,0.,-10.));
#19835=CARTESIAN_POINT('',(-31.1192710879259,-3.81101157296272E-15,-10.));
#19836=CARTESIAN_POINT('Origin',(0.,0.,-10.));
#19837=CARTESIAN_POINT('Origin',(0.,0.,-8.59005579668777));
#19838=CARTESIAN_POINT('',(-31.1192710879259,-3.81101157296272E-15,-7.18011159337554));
#19839=CARTESIAN_POINT('Origin',(0.,0.,-7.18011159337554));
#19840=CARTESIAN_POINT('',(-31.1192710879259,-3.81101157296272E-15,-8.59005579668777));
#19841=CARTESIAN_POINT('Origin',(29.0578798664922,0.,-7.18011159337554));
#19842=CARTESIAN_POINT('',(-29.0578798664922,-3.5585639568508E-15,-7.18011159337554));
#19843=CARTESIAN_POINT('Origin',(0.,0.,-7.18011159337554));
#19844=CARTESIAN_POINT('Origin',(0.,0.,-6.42664169815681));
#19845=CARTESIAN_POINT('',(-29.0578798664922,-3.5585639568508E-15,-5.67317180293808));
#19846=CARTESIAN_POINT('Origin',(0.,0.,-5.67317180293808));
#19847=CARTESIAN_POINT('',(-29.0578798664922,-3.5585639568508E-15,-6.42664169815681));
#19848=CARTESIAN_POINT('Origin',(27.4027293621977,0.,-5.67317180293808));
#19867=UNCERTAINTY_MEASURE_WITH_UNIT(LENGTH_MEASURE(0.01),#19879,
'DISTANCE_ACCURACY_VALUE',
'Maximum model space distance between geometric entities at asserted c
onnectivities');
#19869=UNCERTAINTY_MEASURE_WITH_UNIT(LENGTH_MEASURE(0.01),#19879,
'DISTANCE_ACCURACY_VALUE',
'Maximum model space distance between geometric entities at asserted c
onnectivities');
#19876=(
GEOMETRIC_REPRESENTATION_CONTEXT(3)
GLOBAL_UNCERTAINTY_ASSIGNED_CONTEXT((#19867))
GLOBAL_UNIT_ASSIGNED_CONTEXT((#19879,#19881,#19882))
REPRESENTATION_CONTEXT('','3D')
);
#19878=(
GEOMETRIC_REPRESENTATION_CONTEXT(3)
GLOBAL_UNCERTAINTY_ASSIGNED_CONTEXT((#19869))
GLOBAL_UNIT_ASSIGNED_CONTEXT((#19879,#19881,#19882))
REPRESENTATION_CONTEXT('','3D')
);
#19879=(
LENGTH_UNIT()
NAMED_UNIT(*)
SI_UNIT(.MILLI.,.METRE.)
);
#19881=(
NAMED_UNIT(*)
PLANE_ANGLE_UNIT()
SI_UNIT($,.RADIAN.)
);
#19882=(
NAMED_UNIT(*)
SI_UNIT($,.STERADIAN.)
SOLID_ANGLE_UNIT()
);
#19889=SHAPE_DEFINITION_REPRESENTATION(#19897,#19912);
#19897=PRODUCT_DEFINITION_SHAPE('',$,#19921);
#19912=SHAPE_REPRESENTATION('',(#5309),#19876);
#19914=PRODUCT_DEFINITION_CONTEXT('part definition',#19940,'design');
#19921=PRODUCT_DEFINITION('base','Base',#19929,#19914);
#19929=PRODUCT_DEFINITION_FORMATION('',$,#19948);
#19940=APPLICATION_CONTEXT(
'Core Data for Automotive Mechanical Design Process');
#19941=PRODUCT_CONTEXT('part definition',#19940,'mechanical');
#19948=PRODUCT('base','Base',$,(#19941));
#19951=PRESENTATION_STYLE_ASSIGNMENT((#19957));
#19957=SURFACE_STYLE_USAGE(.BOTH.,#19963);
#19963=SURFACE_SIDE_STYLE('',(#19969));
#19969=SURFACE_STYLE_FILL_AREA(#19975);
#19975=FILL_AREA_STYLE('Opaque(203,203,203)',(#19981));
#19981=FILL_AREA_STYLE_COLOUR('Opaque(203,203,203)',#19987);
#19987=COLOUR_RGB('Opaque(203,203,203)', 0.09019608, 0.27058824, 0.51372549);
ENDSEC;
END-ISO-10303-21;
